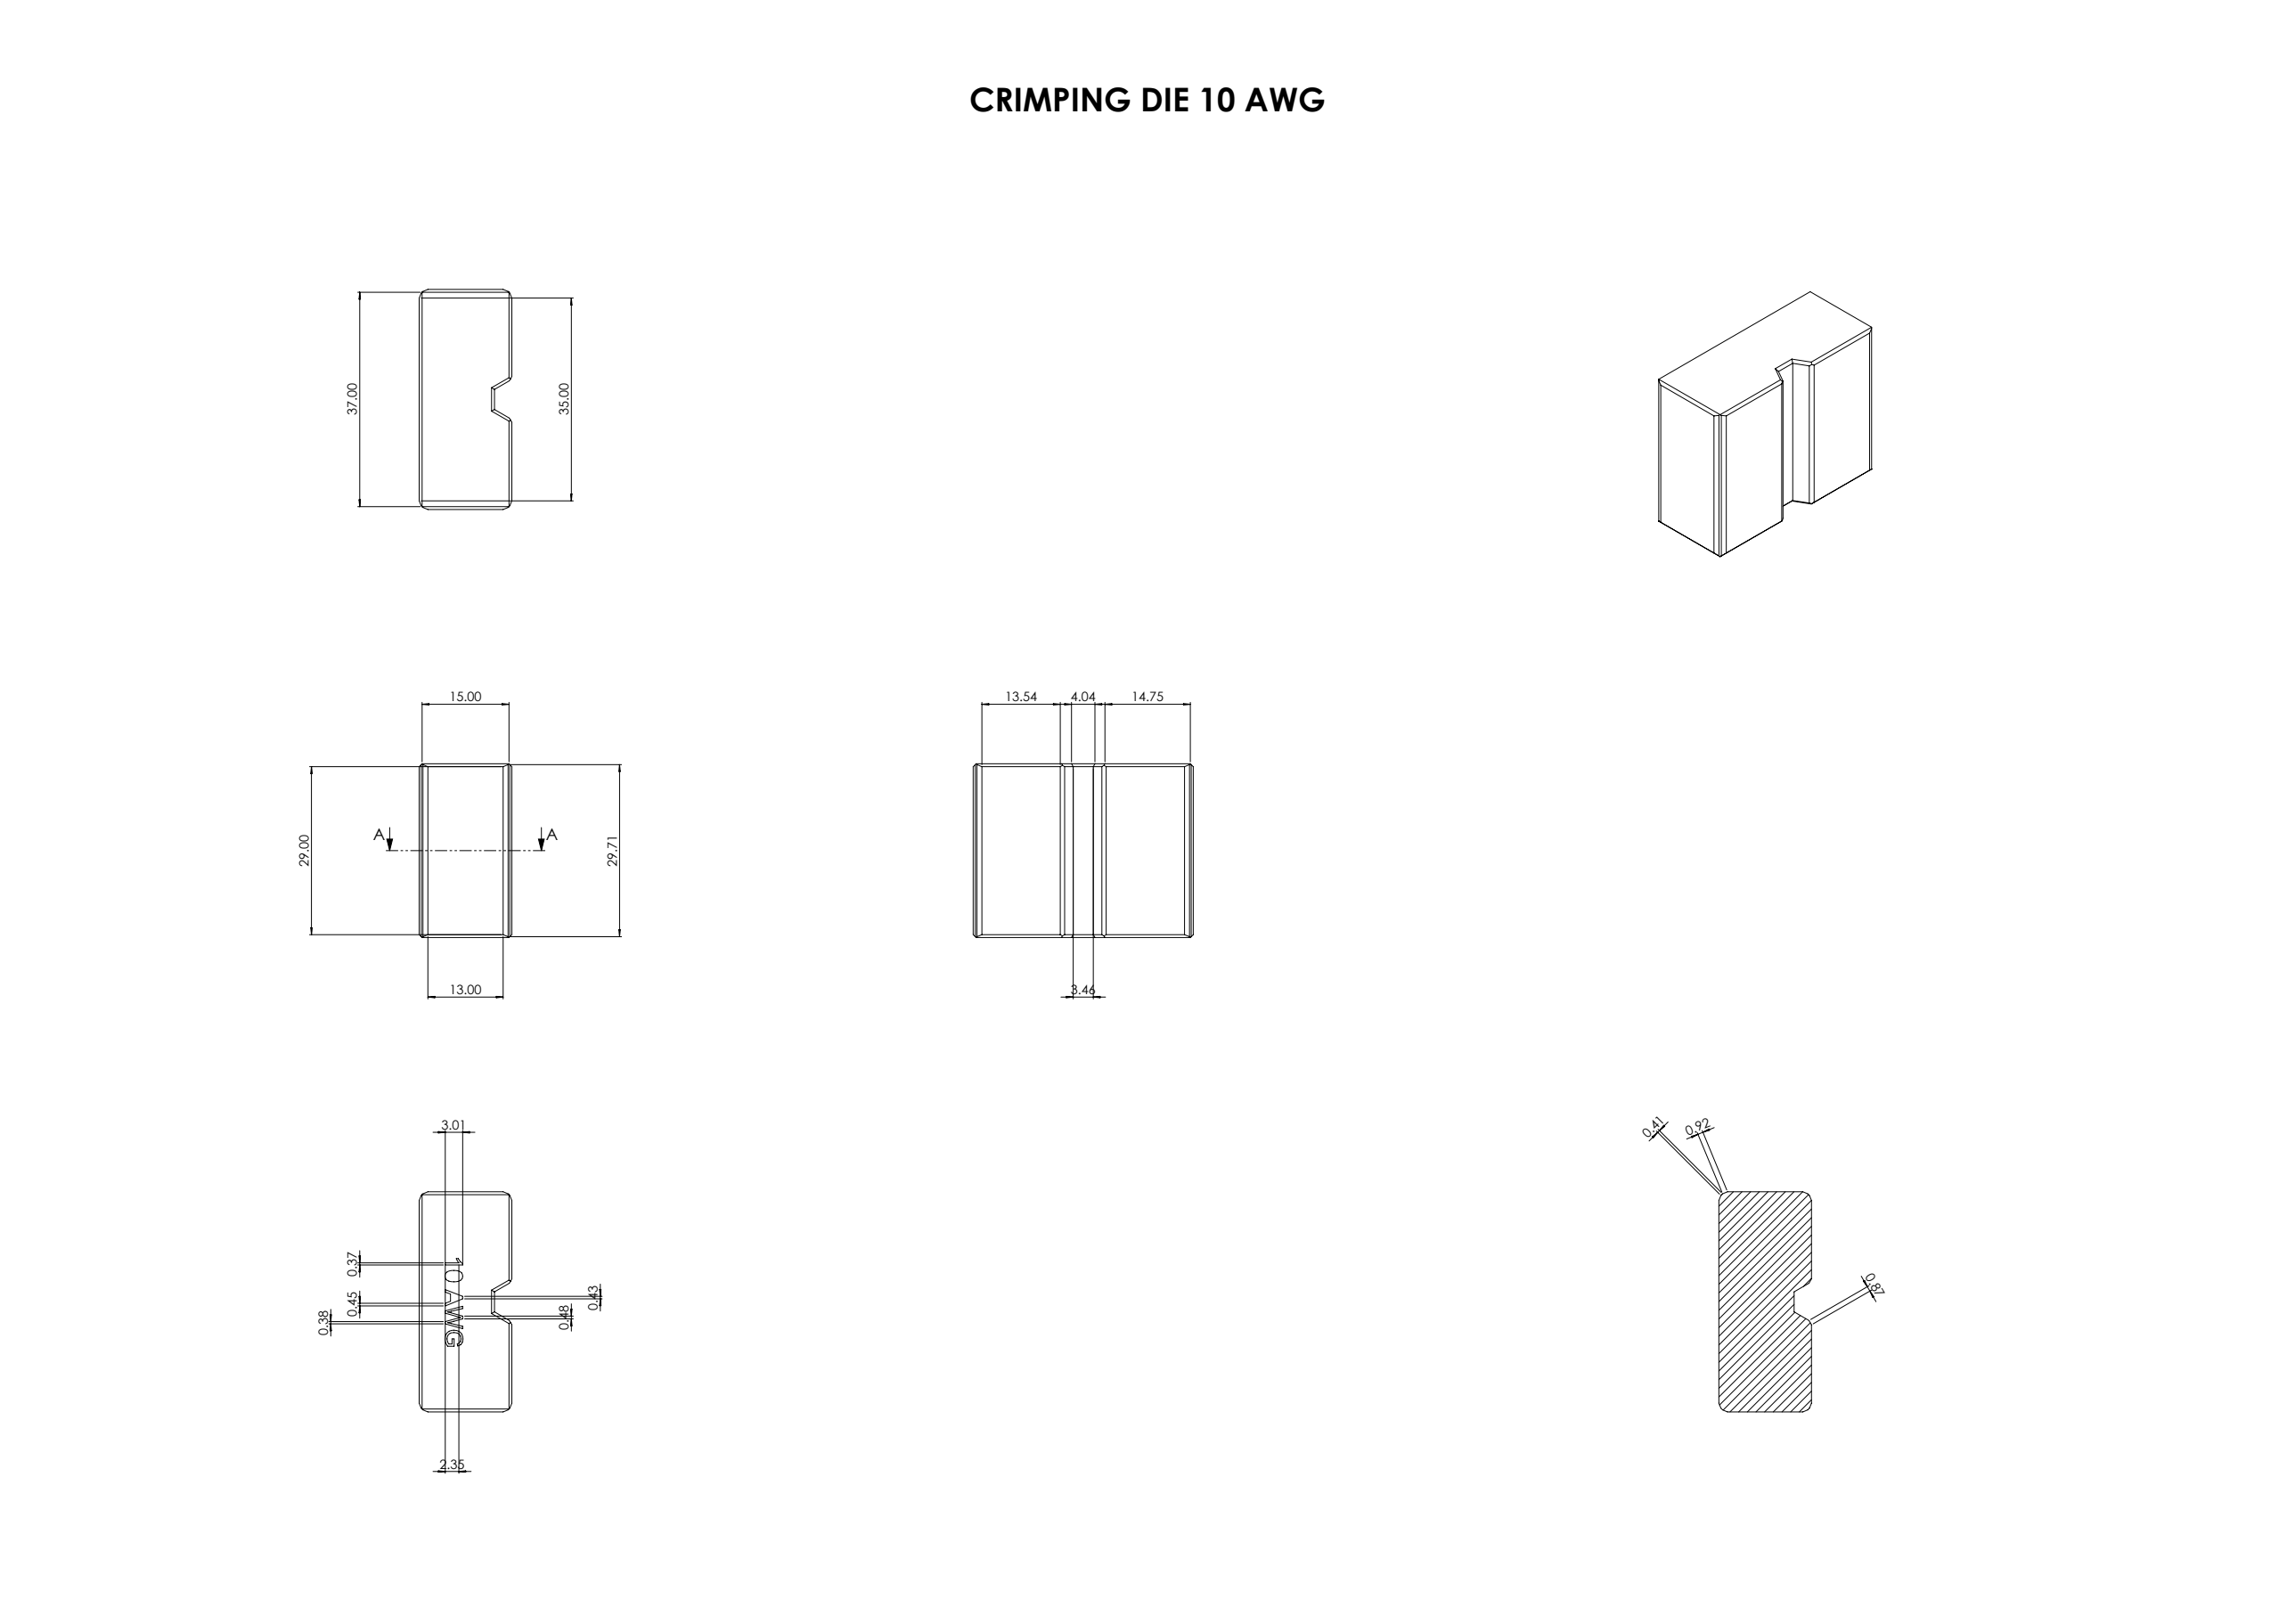
ISO-10303-21;
HEADER;
/* Generated by software containing ST-Developer
 * from STEP Tools, Inc. (www.steptools.com) 
 */

FILE_DESCRIPTION(
/* description */ (''),
/* implementation_level */ '2;1');

FILE_NAME(
/* name */ '08_Crimping_Die_10_AWG.step',
/* time_stamp */ '2026-10-26T03:55:20-07:00',
/* author */ (''),
/* organization */ (''),
/* preprocessor_version */ 'ST-DEVELOPER v20.2',
/* originating_system */ 'Autodesk Translation Framework v15.15.0.0',
/* authorisation */ '');

FILE_SCHEMA (('AUTOMOTIVE_DESIGN { 1 0 10303 214 3 1 1 }'));
ENDSEC;

DATA;
#10=MECHANICAL_DESIGN_GEOMETRIC_PRESENTATION_REPRESENTATION('',(#182),#45236);
#142=SHAPE_REPRESENTATION_RELATIONSHIP('SRR','None',#45321,#162);
#162=ADVANCED_BREP_SHAPE_REPRESENTATION('',(#202),#45223);
#182=STYLED_ITEM('',(#45477),#202);
#202=MANIFOLD_SOLID_BREP('Body1',#16524);
#485=B_SPLINE_CURVE_WITH_KNOTS('',2,(#32438,#32439,#32440),
 .UNSPECIFIED.,.F.,.F.,(3,3),(0.,1.),.UNSPECIFIED.);
#486=B_SPLINE_CURVE_WITH_KNOTS('',2,(#32452,#32453,#32454),
 .UNSPECIFIED.,.F.,.F.,(3,3),(0.,1.),.UNSPECIFIED.);
#487=B_SPLINE_CURVE_WITH_KNOTS('',2,(#32456,#32457,#32458),
 .UNSPECIFIED.,.F.,.F.,(3,3),(0.,1.),.UNSPECIFIED.);
#488=B_SPLINE_CURVE_WITH_KNOTS('',2,(#32466,#32467,#32468),
 .UNSPECIFIED.,.F.,.F.,(3,3),(0.,1.),.UNSPECIFIED.);
#489=B_SPLINE_CURVE_WITH_KNOTS('',2,(#32470,#32471,#32472),
 .UNSPECIFIED.,.F.,.F.,(3,3),(0.,1.),.UNSPECIFIED.);
#490=B_SPLINE_CURVE_WITH_KNOTS('',2,(#32483,#32484,#32485),
 .UNSPECIFIED.,.F.,.F.,(3,3),(0.,1.),.UNSPECIFIED.);
#491=B_SPLINE_CURVE_WITH_KNOTS('',2,(#32504,#32505,#32506),
 .UNSPECIFIED.,.F.,.F.,(3,3),(0.,1.),.UNSPECIFIED.);
#492=B_SPLINE_CURVE_WITH_KNOTS('',2,(#32508,#32509,#32510),
 .UNSPECIFIED.,.F.,.F.,(3,3),(0.,1.),.UNSPECIFIED.);
#493=B_SPLINE_CURVE_WITH_KNOTS('',2,(#32512,#32513,#32514),
 .UNSPECIFIED.,.F.,.F.,(3,3),(0.,1.),.UNSPECIFIED.);
#494=B_SPLINE_CURVE_WITH_KNOTS('',2,(#32516,#32517,#32518),
 .UNSPECIFIED.,.F.,.F.,(3,3),(0.,1.),.UNSPECIFIED.);
#495=B_SPLINE_CURVE_WITH_KNOTS('',2,(#32520,#32521,#32522),
 .UNSPECIFIED.,.F.,.F.,(3,3),(0.,1.),.UNSPECIFIED.);
#496=B_SPLINE_CURVE_WITH_KNOTS('',2,(#32524,#32525,#32526),
 .UNSPECIFIED.,.F.,.F.,(3,3),(0.,1.),.UNSPECIFIED.);
#497=B_SPLINE_CURVE_WITH_KNOTS('',2,(#32528,#32529,#32530),
 .UNSPECIFIED.,.F.,.F.,(3,3),(0.,1.),.UNSPECIFIED.);
#498=B_SPLINE_CURVE_WITH_KNOTS('',2,(#32532,#32533,#32534),
 .UNSPECIFIED.,.F.,.F.,(3,3),(0.,1.),.UNSPECIFIED.);
#499=B_SPLINE_CURVE_WITH_KNOTS('',2,(#32536,#32537,#32538),
 .UNSPECIFIED.,.F.,.F.,(3,3),(0.,1.),.UNSPECIFIED.);
#500=B_SPLINE_CURVE_WITH_KNOTS('',2,(#32540,#32541,#32542),
 .UNSPECIFIED.,.F.,.F.,(3,3),(0.,1.),.UNSPECIFIED.);
#501=B_SPLINE_CURVE_WITH_KNOTS('',2,(#32544,#32545,#32546),
 .UNSPECIFIED.,.F.,.F.,(3,3),(0.,1.),.UNSPECIFIED.);
#502=B_SPLINE_CURVE_WITH_KNOTS('',2,(#32547,#32548,#32549),
 .UNSPECIFIED.,.F.,.F.,(3,3),(0.,1.),.UNSPECIFIED.);
#503=B_SPLINE_CURVE_WITH_KNOTS('',2,(#32552,#32553,#32554),
 .UNSPECIFIED.,.F.,.F.,(3,3),(0.,1.),.UNSPECIFIED.);
#504=B_SPLINE_CURVE_WITH_KNOTS('',2,(#32564,#32565,#32566),
 .UNSPECIFIED.,.F.,.F.,(3,3),(0.,1.),.UNSPECIFIED.);
#505=B_SPLINE_CURVE_WITH_KNOTS('',2,(#32568,#32569,#32570),
 .UNSPECIFIED.,.F.,.F.,(3,3),(0.,1.),.UNSPECIFIED.);
#506=B_SPLINE_CURVE_WITH_KNOTS('',2,(#32573,#32574,#32575),
 .UNSPECIFIED.,.F.,.F.,(3,3),(0.,1.),.UNSPECIFIED.);
#507=B_SPLINE_CURVE_WITH_KNOTS('',2,(#32578,#32579,#32580),
 .UNSPECIFIED.,.F.,.F.,(3,3),(0.,1.),.UNSPECIFIED.);
#508=B_SPLINE_CURVE_WITH_KNOTS('',2,(#32592,#32593,#32594),
 .UNSPECIFIED.,.F.,.F.,(3,3),(0.,1.),.UNSPECIFIED.);
#509=B_SPLINE_CURVE_WITH_KNOTS('',2,(#32596,#32597,#32598),
 .UNSPECIFIED.,.F.,.F.,(3,3),(0.,1.),.UNSPECIFIED.);
#510=B_SPLINE_CURVE_WITH_KNOTS('',2,(#32600,#32601,#32602),
 .UNSPECIFIED.,.F.,.F.,(3,3),(0.,1.),.UNSPECIFIED.);
#511=B_SPLINE_CURVE_WITH_KNOTS('',2,(#32604,#32605,#32606),
 .UNSPECIFIED.,.F.,.F.,(3,3),(0.,1.),.UNSPECIFIED.);
#512=B_SPLINE_CURVE_WITH_KNOTS('',2,(#32608,#32609,#32610),
 .UNSPECIFIED.,.F.,.F.,(3,3),(0.,1.),.UNSPECIFIED.);
#513=B_SPLINE_CURVE_WITH_KNOTS('',2,(#32612,#32613,#32614),
 .UNSPECIFIED.,.F.,.F.,(3,3),(0.,1.),.UNSPECIFIED.);
#514=B_SPLINE_CURVE_WITH_KNOTS('',2,(#32616,#32617,#32618),
 .UNSPECIFIED.,.F.,.F.,(3,3),(0.,1.),.UNSPECIFIED.);
#515=B_SPLINE_CURVE_WITH_KNOTS('',2,(#32620,#32621,#32622),
 .UNSPECIFIED.,.F.,.F.,(3,3),(0.,1.),.UNSPECIFIED.);
#516=B_SPLINE_CURVE_WITH_KNOTS('',2,(#32624,#32625,#32626),
 .UNSPECIFIED.,.F.,.F.,(3,3),(0.,1.),.UNSPECIFIED.);
#517=B_SPLINE_CURVE_WITH_KNOTS('',2,(#32628,#32629,#32630),
 .UNSPECIFIED.,.F.,.F.,(3,3),(0.,1.),.UNSPECIFIED.);
#518=B_SPLINE_CURVE_WITH_KNOTS('',2,(#32632,#32633,#32634),
 .UNSPECIFIED.,.F.,.F.,(3,3),(0.,1.),.UNSPECIFIED.);
#519=B_SPLINE_CURVE_WITH_KNOTS('',2,(#32638,#32639,#32640),
 .UNSPECIFIED.,.F.,.F.,(3,3),(0.,1.),.UNSPECIFIED.);
#520=B_SPLINE_CURVE_WITH_KNOTS('',2,(#32642,#32643,#32644),
 .UNSPECIFIED.,.F.,.F.,(3,3),(0.,1.),.UNSPECIFIED.);
#521=B_SPLINE_CURVE_WITH_KNOTS('',2,(#32646,#32647,#32648),
 .UNSPECIFIED.,.F.,.F.,(3,3),(0.,1.),.UNSPECIFIED.);
#522=B_SPLINE_CURVE_WITH_KNOTS('',2,(#32650,#32651,#32652),
 .UNSPECIFIED.,.F.,.F.,(3,3),(0.,1.),.UNSPECIFIED.);
#523=B_SPLINE_CURVE_WITH_KNOTS('',2,(#32654,#32655,#32656),
 .UNSPECIFIED.,.F.,.F.,(3,3),(0.,1.),.UNSPECIFIED.);
#524=B_SPLINE_CURVE_WITH_KNOTS('',2,(#32658,#32659,#32660),
 .UNSPECIFIED.,.F.,.F.,(3,3),(0.,1.),.UNSPECIFIED.);
#525=B_SPLINE_CURVE_WITH_KNOTS('',2,(#32662,#32663,#32664),
 .UNSPECIFIED.,.F.,.F.,(3,3),(0.,1.),.UNSPECIFIED.);
#526=B_SPLINE_CURVE_WITH_KNOTS('',2,(#32666,#32667,#32668),
 .UNSPECIFIED.,.F.,.F.,(3,3),(0.,1.),.UNSPECIFIED.);
#527=B_SPLINE_CURVE_WITH_KNOTS('',2,(#32670,#32671,#32672),
 .UNSPECIFIED.,.F.,.F.,(3,3),(0.,1.),.UNSPECIFIED.);
#528=B_SPLINE_CURVE_WITH_KNOTS('',2,(#32674,#32675,#32676),
 .UNSPECIFIED.,.F.,.F.,(3,3),(0.,1.),.UNSPECIFIED.);
#529=B_SPLINE_CURVE_WITH_KNOTS('',2,(#32677,#32678,#32679),
 .UNSPECIFIED.,.F.,.F.,(3,3),(0.,1.),.UNSPECIFIED.);
#530=B_SPLINE_CURVE_WITH_KNOTS('',2,(#32712,#32713,#32714),
 .UNSPECIFIED.,.F.,.F.,(3,3),(0.,1.),.UNSPECIFIED.);
#531=B_SPLINE_CURVE_WITH_KNOTS('',2,(#32724,#32725,#32726),
 .UNSPECIFIED.,.F.,.F.,(3,3),(0.,1.),.UNSPECIFIED.);
#532=B_SPLINE_CURVE_WITH_KNOTS('',2,(#32755,#32756,#32757),
 .UNSPECIFIED.,.F.,.F.,(3,3),(0.,1.),.UNSPECIFIED.);
#533=B_SPLINE_CURVE_WITH_KNOTS('',2,(#32766,#32767,#32768),
 .UNSPECIFIED.,.F.,.F.,(3,3),(0.,1.),.UNSPECIFIED.);
#534=B_SPLINE_CURVE_WITH_KNOTS('',2,(#32789,#32790,#32791),
 .UNSPECIFIED.,.F.,.F.,(3,3),(0.,1.),.UNSPECIFIED.);
#535=B_SPLINE_CURVE_WITH_KNOTS('',2,(#32800,#32801,#32802),
 .UNSPECIFIED.,.F.,.F.,(3,3),(0.,1.),.UNSPECIFIED.);
#536=B_SPLINE_CURVE_WITH_KNOTS('',2,(#32864,#32865,#32866),
 .UNSPECIFIED.,.F.,.F.,(3,3),(0.,1.),.UNSPECIFIED.);
#537=B_SPLINE_CURVE_WITH_KNOTS('',2,(#32876,#32877,#32878),
 .UNSPECIFIED.,.F.,.F.,(3,3),(0.,1.),.UNSPECIFIED.);
#538=B_SPLINE_CURVE_WITH_KNOTS('',2,(#32887,#32888,#32889),
 .UNSPECIFIED.,.F.,.F.,(3,3),(0.,1.),.UNSPECIFIED.);
#539=B_SPLINE_CURVE_WITH_KNOTS('',2,(#32898,#32899,#32900),
 .UNSPECIFIED.,.F.,.F.,(3,3),(0.,1.),.UNSPECIFIED.);
#540=B_SPLINE_CURVE_WITH_KNOTS('',2,(#32909,#32910,#32911),
 .UNSPECIFIED.,.F.,.F.,(3,3),(0.,1.),.UNSPECIFIED.);
#541=B_SPLINE_CURVE_WITH_KNOTS('',2,(#32920,#32921,#32922),
 .UNSPECIFIED.,.F.,.F.,(3,3),(0.,1.),.UNSPECIFIED.);
#542=B_SPLINE_CURVE_WITH_KNOTS('',2,(#32931,#32932,#32933),
 .UNSPECIFIED.,.F.,.F.,(3,3),(0.,1.),.UNSPECIFIED.);
#543=B_SPLINE_CURVE_WITH_KNOTS('',2,(#32942,#32943,#32944),
 .UNSPECIFIED.,.F.,.F.,(3,3),(0.,1.),.UNSPECIFIED.);
#544=B_SPLINE_CURVE_WITH_KNOTS('',2,(#32953,#32954,#32955),
 .UNSPECIFIED.,.F.,.F.,(3,3),(0.,1.),.UNSPECIFIED.);
#545=B_SPLINE_CURVE_WITH_KNOTS('',2,(#32964,#32965,#32966),
 .UNSPECIFIED.,.F.,.F.,(3,3),(0.,1.),.UNSPECIFIED.);
#546=B_SPLINE_CURVE_WITH_KNOTS('',2,(#32975,#32976,#32977),
 .UNSPECIFIED.,.F.,.F.,(3,3),(0.,1.),.UNSPECIFIED.);
#547=B_SPLINE_CURVE_WITH_KNOTS('',2,(#32984,#32985,#32986),
 .UNSPECIFIED.,.F.,.F.,(3,3),(0.,1.),.UNSPECIFIED.);
#548=B_SPLINE_CURVE_WITH_KNOTS('',2,(#32997,#32998,#32999),
 .UNSPECIFIED.,.F.,.F.,(3,3),(0.,1.),.UNSPECIFIED.);
#549=B_SPLINE_CURVE_WITH_KNOTS('',2,(#33009,#33010,#33011),
 .UNSPECIFIED.,.F.,.F.,(3,3),(0.,1.),.UNSPECIFIED.);
#550=B_SPLINE_CURVE_WITH_KNOTS('',2,(#33024,#33025,#33026),
 .UNSPECIFIED.,.F.,.F.,(3,3),(0.,1.),.UNSPECIFIED.);
#551=B_SPLINE_CURVE_WITH_KNOTS('',2,(#33035,#33036,#33037),
 .UNSPECIFIED.,.F.,.F.,(3,3),(0.,1.),.UNSPECIFIED.);
#552=B_SPLINE_CURVE_WITH_KNOTS('',2,(#33062,#33063,#33064),
 .UNSPECIFIED.,.F.,.F.,(3,3),(0.,1.),.UNSPECIFIED.);
#553=B_SPLINE_CURVE_WITH_KNOTS('',2,(#33074,#33075,#33076),
 .UNSPECIFIED.,.F.,.F.,(3,3),(0.,1.),.UNSPECIFIED.);
#554=B_SPLINE_CURVE_WITH_KNOTS('',2,(#33085,#33086,#33087),
 .UNSPECIFIED.,.F.,.F.,(3,3),(0.,1.),.UNSPECIFIED.);
#555=B_SPLINE_CURVE_WITH_KNOTS('',2,(#33096,#33097,#33098),
 .UNSPECIFIED.,.F.,.F.,(3,3),(0.,1.),.UNSPECIFIED.);
#556=B_SPLINE_CURVE_WITH_KNOTS('',2,(#33107,#33108,#33109),
 .UNSPECIFIED.,.F.,.F.,(3,3),(0.,1.),.UNSPECIFIED.);
#557=B_SPLINE_CURVE_WITH_KNOTS('',2,(#33118,#33119,#33120),
 .UNSPECIFIED.,.F.,.F.,(3,3),(0.,1.),.UNSPECIFIED.);
#558=B_SPLINE_CURVE_WITH_KNOTS('',2,(#33129,#33130,#33131),
 .UNSPECIFIED.,.F.,.F.,(3,3),(0.,1.),.UNSPECIFIED.);
#559=B_SPLINE_CURVE_WITH_KNOTS('',2,(#33140,#33141,#33142),
 .UNSPECIFIED.,.F.,.F.,(3,3),(0.,1.),.UNSPECIFIED.);
#560=B_SPLINE_CURVE_WITH_KNOTS('',2,(#33151,#33152,#33153),
 .UNSPECIFIED.,.F.,.F.,(3,3),(0.,1.),.UNSPECIFIED.);
#561=B_SPLINE_CURVE_WITH_KNOTS('',2,(#33162,#33163,#33164),
 .UNSPECIFIED.,.F.,.F.,(3,3),(0.,1.),.UNSPECIFIED.);
#562=B_SPLINE_CURVE_WITH_KNOTS('',2,(#33173,#33174,#33175),
 .UNSPECIFIED.,.F.,.F.,(3,3),(0.,1.),.UNSPECIFIED.);
#563=B_SPLINE_CURVE_WITH_KNOTS('',2,(#33184,#33185,#33186),
 .UNSPECIFIED.,.F.,.F.,(3,3),(0.,1.),.UNSPECIFIED.);
#564=B_SPLINE_CURVE_WITH_KNOTS('',2,(#33199,#33200,#33201),
 .UNSPECIFIED.,.F.,.F.,(3,3),(0.,1.),.UNSPECIFIED.);
#565=B_SPLINE_CURVE_WITH_KNOTS('',2,(#33210,#33211,#33212),
 .UNSPECIFIED.,.F.,.F.,(3,3),(0.,1.),.UNSPECIFIED.);
#566=B_SPLINE_CURVE_WITH_KNOTS('',2,(#33221,#33222,#33223),
 .UNSPECIFIED.,.F.,.F.,(3,3),(0.,1.),.UNSPECIFIED.);
#567=B_SPLINE_CURVE_WITH_KNOTS('',2,(#33232,#33233,#33234),
 .UNSPECIFIED.,.F.,.F.,(3,3),(0.,1.),.UNSPECIFIED.);
#568=B_SPLINE_CURVE_WITH_KNOTS('',2,(#33243,#33244,#33245),
 .UNSPECIFIED.,.F.,.F.,(3,3),(0.,1.),.UNSPECIFIED.);
#569=B_SPLINE_CURVE_WITH_KNOTS('',2,(#33254,#33255,#33256),
 .UNSPECIFIED.,.F.,.F.,(3,3),(0.,1.),.UNSPECIFIED.);
#570=B_SPLINE_CURVE_WITH_KNOTS('',2,(#33265,#33266,#33267),
 .UNSPECIFIED.,.F.,.F.,(3,3),(0.,1.),.UNSPECIFIED.);
#571=B_SPLINE_CURVE_WITH_KNOTS('',2,(#33276,#33277,#33278),
 .UNSPECIFIED.,.F.,.F.,(3,3),(0.,1.),.UNSPECIFIED.);
#572=B_SPLINE_CURVE_WITH_KNOTS('',2,(#33287,#33288,#33289),
 .UNSPECIFIED.,.F.,.F.,(3,3),(0.,1.),.UNSPECIFIED.);
#573=B_SPLINE_CURVE_WITH_KNOTS('',2,(#33298,#33299,#33300),
 .UNSPECIFIED.,.F.,.F.,(3,3),(0.,1.),.UNSPECIFIED.);
#574=B_SPLINE_CURVE_WITH_KNOTS('',2,(#33309,#33310,#33311),
 .UNSPECIFIED.,.F.,.F.,(3,3),(0.,1.),.UNSPECIFIED.);
#858=B_SPLINE_SURFACE_WITH_KNOTS('',2,1,((#32703,#32704),(#32705,#32706),
(#32707,#32708)),.UNSPECIFIED.,.F.,.F.,.F.,(3,3),(2,2),(0.,1.),(0.,0.0249999999999999),
 .UNSPECIFIED.);
#859=B_SPLINE_SURFACE_WITH_KNOTS('',2,1,((#32716,#32717),(#32718,#32719),
(#32720,#32721)),.UNSPECIFIED.,.F.,.F.,.F.,(3,3),(2,2),(0.,1.),(0.,0.0249999999999999),
 .UNSPECIFIED.);
#860=B_SPLINE_SURFACE_WITH_KNOTS('',2,1,((#32747,#32748),(#32749,#32750),
(#32751,#32752)),.UNSPECIFIED.,.F.,.F.,.F.,(3,3),(2,2),(0.,1.),(0.,0.0249999999999999),
 .UNSPECIFIED.);
#861=B_SPLINE_SURFACE_WITH_KNOTS('',2,1,((#32758,#32759),(#32760,#32761),
(#32762,#32763)),.UNSPECIFIED.,.F.,.F.,.F.,(3,3),(2,2),(0.,1.),(0.,0.0249999999999999),
 .UNSPECIFIED.);
#862=B_SPLINE_SURFACE_WITH_KNOTS('',2,1,((#32781,#32782),(#32783,#32784),
(#32785,#32786)),.UNSPECIFIED.,.F.,.F.,.F.,(3,3),(2,2),(0.,1.),(0.,0.0249999999999999),
 .UNSPECIFIED.);
#863=B_SPLINE_SURFACE_WITH_KNOTS('',2,1,((#32792,#32793),(#32794,#32795),
(#32796,#32797)),.UNSPECIFIED.,.F.,.F.,.F.,(3,3),(2,2),(0.,1.),(0.,0.0249999999999999),
 .UNSPECIFIED.);
#864=B_SPLINE_SURFACE_WITH_KNOTS('',2,1,((#32855,#32856),(#32857,#32858),
(#32859,#32860)),.UNSPECIFIED.,.F.,.F.,.F.,(3,3),(2,2),(0.,1.),(0.,0.0249999999999999),
 .UNSPECIFIED.);
#865=B_SPLINE_SURFACE_WITH_KNOTS('',2,1,((#32868,#32869),(#32870,#32871),
(#32872,#32873)),.UNSPECIFIED.,.F.,.F.,.F.,(3,3),(2,2),(0.,1.),(0.,0.0249999999999999),
 .UNSPECIFIED.);
#866=B_SPLINE_SURFACE_WITH_KNOTS('',2,1,((#32879,#32880),(#32881,#32882),
(#32883,#32884)),.UNSPECIFIED.,.F.,.F.,.F.,(3,3),(2,2),(0.,1.),(0.,0.0249999999999999),
 .UNSPECIFIED.);
#867=B_SPLINE_SURFACE_WITH_KNOTS('',2,1,((#32890,#32891),(#32892,#32893),
(#32894,#32895)),.UNSPECIFIED.,.F.,.F.,.F.,(3,3),(2,2),(0.,1.),(0.,0.0249999999999999),
 .UNSPECIFIED.);
#868=B_SPLINE_SURFACE_WITH_KNOTS('',2,1,((#32901,#32902),(#32903,#32904),
(#32905,#32906)),.UNSPECIFIED.,.F.,.F.,.F.,(3,3),(2,2),(0.,1.),(0.,0.0249999999999999),
 .UNSPECIFIED.);
#869=B_SPLINE_SURFACE_WITH_KNOTS('',2,1,((#32912,#32913),(#32914,#32915),
(#32916,#32917)),.UNSPECIFIED.,.F.,.F.,.F.,(3,3),(2,2),(0.,1.),(0.,0.0249999999999999),
 .UNSPECIFIED.);
#870=B_SPLINE_SURFACE_WITH_KNOTS('',2,1,((#32923,#32924),(#32925,#32926),
(#32927,#32928)),.UNSPECIFIED.,.F.,.F.,.F.,(3,3),(2,2),(0.,1.),(0.,0.0249999999999999),
 .UNSPECIFIED.);
#871=B_SPLINE_SURFACE_WITH_KNOTS('',2,1,((#32934,#32935),(#32936,#32937),
(#32938,#32939)),.UNSPECIFIED.,.F.,.F.,.F.,(3,3),(2,2),(0.,1.),(0.,0.0249999999999999),
 .UNSPECIFIED.);
#872=B_SPLINE_SURFACE_WITH_KNOTS('',2,1,((#32945,#32946),(#32947,#32948),
(#32949,#32950)),.UNSPECIFIED.,.F.,.F.,.F.,(3,3),(2,2),(0.,1.),(0.,0.0249999999999999),
 .UNSPECIFIED.);
#873=B_SPLINE_SURFACE_WITH_KNOTS('',2,1,((#32956,#32957),(#32958,#32959),
(#32960,#32961)),.UNSPECIFIED.,.F.,.F.,.F.,(3,3),(2,2),(0.,1.),(0.,0.0249999999999999),
 .UNSPECIFIED.);
#874=B_SPLINE_SURFACE_WITH_KNOTS('',2,1,((#32967,#32968),(#32969,#32970),
(#32971,#32972)),.UNSPECIFIED.,.F.,.F.,.F.,(3,3),(2,2),(0.,1.),(0.,0.0249999999999999),
 .UNSPECIFIED.);
#875=B_SPLINE_SURFACE_WITH_KNOTS('',2,1,((#32978,#32979),(#32980,#32981),
(#32982,#32983)),.UNSPECIFIED.,.F.,.F.,.F.,(3,3),(2,2),(0.,1.),(0.,0.0249999999999999),
 .UNSPECIFIED.);
#876=B_SPLINE_SURFACE_WITH_KNOTS('',2,1,((#32988,#32989),(#32990,#32991),
(#32992,#32993)),.UNSPECIFIED.,.F.,.F.,.F.,(3,3),(2,2),(0.,1.),(0.,0.0249999999999999),
 .UNSPECIFIED.);
#877=B_SPLINE_SURFACE_WITH_KNOTS('',2,1,((#33001,#33002),(#33003,#33004),
(#33005,#33006)),.UNSPECIFIED.,.F.,.F.,.F.,(3,3),(2,2),(0.,1.),(0.,0.0249999999999999),
 .UNSPECIFIED.);
#878=B_SPLINE_SURFACE_WITH_KNOTS('',2,1,((#33016,#33017),(#33018,#33019),
(#33020,#33021)),.UNSPECIFIED.,.F.,.F.,.F.,(3,3),(2,2),(0.,1.),(0.,0.0249999999999999),
 .UNSPECIFIED.);
#879=B_SPLINE_SURFACE_WITH_KNOTS('',2,1,((#33027,#33028),(#33029,#33030),
(#33031,#33032)),.UNSPECIFIED.,.F.,.F.,.F.,(3,3),(2,2),(0.,1.),(0.,0.0249999999999999),
 .UNSPECIFIED.);
#880=B_SPLINE_SURFACE_WITH_KNOTS('',2,1,((#33053,#33054),(#33055,#33056),
(#33057,#33058)),.UNSPECIFIED.,.F.,.F.,.F.,(3,3),(2,2),(0.,1.),(0.,0.0249999999999999),
 .UNSPECIFIED.);
#881=B_SPLINE_SURFACE_WITH_KNOTS('',2,1,((#33066,#33067),(#33068,#33069),
(#33070,#33071)),.UNSPECIFIED.,.F.,.F.,.F.,(3,3),(2,2),(0.,1.),(0.,0.0249999999999999),
 .UNSPECIFIED.);
#882=B_SPLINE_SURFACE_WITH_KNOTS('',2,1,((#33077,#33078),(#33079,#33080),
(#33081,#33082)),.UNSPECIFIED.,.F.,.F.,.F.,(3,3),(2,2),(0.,1.),(0.,0.0249999999999999),
 .UNSPECIFIED.);
#883=B_SPLINE_SURFACE_WITH_KNOTS('',2,1,((#33088,#33089),(#33090,#33091),
(#33092,#33093)),.UNSPECIFIED.,.F.,.F.,.F.,(3,3),(2,2),(0.,1.),(0.,0.0249999999999999),
 .UNSPECIFIED.);
#884=B_SPLINE_SURFACE_WITH_KNOTS('',2,1,((#33099,#33100),(#33101,#33102),
(#33103,#33104)),.UNSPECIFIED.,.F.,.F.,.F.,(3,3),(2,2),(0.,1.),(0.,0.0249999999999999),
 .UNSPECIFIED.);
#885=B_SPLINE_SURFACE_WITH_KNOTS('',2,1,((#33110,#33111),(#33112,#33113),
(#33114,#33115)),.UNSPECIFIED.,.F.,.F.,.F.,(3,3),(2,2),(0.,1.),(0.,0.0249999999999999),
 .UNSPECIFIED.);
#886=B_SPLINE_SURFACE_WITH_KNOTS('',2,1,((#33121,#33122),(#33123,#33124),
(#33125,#33126)),.UNSPECIFIED.,.F.,.F.,.F.,(3,3),(2,2),(0.,1.),(0.,0.0249999999999999),
 .UNSPECIFIED.);
#887=B_SPLINE_SURFACE_WITH_KNOTS('',2,1,((#33132,#33133),(#33134,#33135),
(#33136,#33137)),.UNSPECIFIED.,.F.,.F.,.F.,(3,3),(2,2),(0.,1.),(0.,0.0249999999999999),
 .UNSPECIFIED.);
#888=B_SPLINE_SURFACE_WITH_KNOTS('',2,1,((#33143,#33144),(#33145,#33146),
(#33147,#33148)),.UNSPECIFIED.,.F.,.F.,.F.,(3,3),(2,2),(0.,1.),(0.,0.0249999999999999),
 .UNSPECIFIED.);
#889=B_SPLINE_SURFACE_WITH_KNOTS('',2,1,((#33154,#33155),(#33156,#33157),
(#33158,#33159)),.UNSPECIFIED.,.F.,.F.,.F.,(3,3),(2,2),(0.,1.),(0.,0.0249999999999999),
 .UNSPECIFIED.);
#890=B_SPLINE_SURFACE_WITH_KNOTS('',2,1,((#33165,#33166),(#33167,#33168),
(#33169,#33170)),.UNSPECIFIED.,.F.,.F.,.F.,(3,3),(2,2),(0.,1.),(0.,0.0249999999999999),
 .UNSPECIFIED.);
#891=B_SPLINE_SURFACE_WITH_KNOTS('',2,1,((#33176,#33177),(#33178,#33179),
(#33180,#33181)),.UNSPECIFIED.,.F.,.F.,.F.,(3,3),(2,2),(0.,1.),(0.,0.0249999999999999),
 .UNSPECIFIED.);
#892=B_SPLINE_SURFACE_WITH_KNOTS('',2,1,((#33191,#33192),(#33193,#33194),
(#33195,#33196)),.UNSPECIFIED.,.F.,.F.,.F.,(3,3),(2,2),(0.,1.),(0.,0.0249999999999999),
 .UNSPECIFIED.);
#893=B_SPLINE_SURFACE_WITH_KNOTS('',2,1,((#33202,#33203),(#33204,#33205),
(#33206,#33207)),.UNSPECIFIED.,.F.,.F.,.F.,(3,3),(2,2),(0.,1.),(0.,0.0249999999999999),
 .UNSPECIFIED.);
#894=B_SPLINE_SURFACE_WITH_KNOTS('',2,1,((#33213,#33214),(#33215,#33216),
(#33217,#33218)),.UNSPECIFIED.,.F.,.F.,.F.,(3,3),(2,2),(0.,1.),(0.,0.0249999999999999),
 .UNSPECIFIED.);
#895=B_SPLINE_SURFACE_WITH_KNOTS('',2,1,((#33224,#33225),(#33226,#33227),
(#33228,#33229)),.UNSPECIFIED.,.F.,.F.,.F.,(3,3),(2,2),(0.,1.),(0.,0.0249999999999999),
 .UNSPECIFIED.);
#896=B_SPLINE_SURFACE_WITH_KNOTS('',2,1,((#33235,#33236),(#33237,#33238),
(#33239,#33240)),.UNSPECIFIED.,.F.,.F.,.F.,(3,3),(2,2),(0.,1.),(0.,0.0249999999999999),
 .UNSPECIFIED.);
#897=B_SPLINE_SURFACE_WITH_KNOTS('',2,1,((#33246,#33247),(#33248,#33249),
(#33250,#33251)),.UNSPECIFIED.,.F.,.F.,.F.,(3,3),(2,2),(0.,1.),(0.,0.0249999999999999),
 .UNSPECIFIED.);
#898=B_SPLINE_SURFACE_WITH_KNOTS('',2,1,((#33257,#33258),(#33259,#33260),
(#33261,#33262)),.UNSPECIFIED.,.F.,.F.,.F.,(3,3),(2,2),(0.,1.),(0.,0.0249999999999999),
 .UNSPECIFIED.);
#899=B_SPLINE_SURFACE_WITH_KNOTS('',2,1,((#33268,#33269),(#33270,#33271),
(#33272,#33273)),.UNSPECIFIED.,.F.,.F.,.F.,(3,3),(2,2),(0.,1.),(0.,0.0249999999999999),
 .UNSPECIFIED.);
#900=B_SPLINE_SURFACE_WITH_KNOTS('',2,1,((#33279,#33280),(#33281,#33282),
(#33283,#33284)),.UNSPECIFIED.,.F.,.F.,.F.,(3,3),(2,2),(0.,1.),(0.,0.0249999999999999),
 .UNSPECIFIED.);
#901=B_SPLINE_SURFACE_WITH_KNOTS('',2,1,((#33290,#33291),(#33292,#33293),
(#33294,#33295)),.UNSPECIFIED.,.F.,.F.,.F.,(3,3),(2,2),(0.,1.),(0.,0.0249999999999999),
 .UNSPECIFIED.);
#902=B_SPLINE_SURFACE_WITH_KNOTS('',2,1,((#33301,#33302),(#33303,#33304),
(#33305,#33306)),.UNSPECIFIED.,.F.,.F.,.F.,(3,3),(2,2),(0.,1.),(0.,0.0249999999999999),
 .UNSPECIFIED.);
#965=FACE_BOUND('',#3127,.T.);
#966=FACE_BOUND('',#3128,.T.);
#967=FACE_BOUND('',#3129,.T.);
#968=FACE_BOUND('',#3130,.T.);
#969=FACE_BOUND('',#3131,.T.);
#1136=PLANE('',#17176);
#1137=PLANE('',#17177);
#1138=PLANE('',#17178);
#1139=PLANE('',#17179);
#1140=PLANE('',#17180);
#1141=PLANE('',#17181);
#1142=PLANE('',#17182);
#1143=PLANE('',#17183);
#1144=PLANE('',#17184);
#1145=PLANE('',#17185);
#1146=PLANE('',#17186);
#1147=PLANE('',#17187);
#1148=PLANE('',#17188);
#1149=PLANE('',#17189);
#1150=PLANE('',#17190);
#1151=PLANE('',#17191);
#1152=PLANE('',#17192);
#1153=PLANE('',#17193);
#1154=PLANE('',#17194);
#1155=PLANE('',#17195);
#1156=PLANE('',#17196);
#1157=PLANE('',#17197);
#1158=PLANE('',#17198);
#1159=PLANE('',#17199);
#1160=PLANE('',#17200);
#1161=PLANE('',#17201);
#1162=PLANE('',#17202);
#1163=PLANE('',#17203);
#1164=PLANE('',#17204);
#1165=PLANE('',#17205);
#1166=PLANE('',#17206);
#1167=PLANE('',#17207);
#1168=PLANE('',#17208);
#1169=PLANE('',#17209);
#1170=PLANE('',#17210);
#1171=PLANE('',#17211);
#1172=PLANE('',#17212);
#1173=PLANE('',#17213);
#1174=PLANE('',#17214);
#1175=PLANE('',#17215);
#1176=PLANE('',#17216);
#1177=PLANE('',#17217);
#1178=PLANE('',#17218);
#1179=PLANE('',#17219);
#1180=PLANE('',#17220);
#1181=PLANE('',#17221);
#1182=PLANE('',#17222);
#1183=PLANE('',#17223);
#1184=PLANE('',#17224);
#1185=PLANE('',#17225);
#1186=PLANE('',#17226);
#1187=PLANE('',#17227);
#1188=PLANE('',#17228);
#1189=PLANE('',#17229);
#1190=PLANE('',#17230);
#1191=PLANE('',#17231);
#1192=PLANE('',#17232);
#1193=PLANE('',#17233);
#1194=PLANE('',#17234);
#1195=PLANE('',#17235);
#1196=PLANE('',#17236);
#1197=PLANE('',#17237);
#1198=PLANE('',#17238);
#1199=PLANE('',#17239);
#1200=PLANE('',#17240);
#1201=PLANE('',#17241);
#1202=PLANE('',#17242);
#1203=PLANE('',#17243);
#1204=PLANE('',#17244);
#1205=PLANE('',#17245);
#1206=PLANE('',#17246);
#1207=PLANE('',#17247);
#1208=PLANE('',#17248);
#1209=PLANE('',#17249);
#1210=PLANE('',#17250);
#1211=PLANE('',#17251);
#1212=PLANE('',#17252);
#2101=FACE_OUTER_BOUND('',#3101,.T.);
#2102=FACE_OUTER_BOUND('',#3102,.T.);
#2103=FACE_OUTER_BOUND('',#3103,.T.);
#2104=FACE_OUTER_BOUND('',#3104,.T.);
#2105=FACE_OUTER_BOUND('',#3105,.T.);
#2106=FACE_OUTER_BOUND('',#3106,.T.);
#2107=FACE_OUTER_BOUND('',#3107,.T.);
#2108=FACE_OUTER_BOUND('',#3108,.T.);
#2109=FACE_OUTER_BOUND('',#3109,.T.);
#2110=FACE_OUTER_BOUND('',#3110,.T.);
#2111=FACE_OUTER_BOUND('',#3111,.T.);
#2112=FACE_OUTER_BOUND('',#3112,.T.);
#2113=FACE_OUTER_BOUND('',#3113,.T.);
#2114=FACE_OUTER_BOUND('',#3114,.T.);
#2115=FACE_OUTER_BOUND('',#3115,.T.);
#2116=FACE_OUTER_BOUND('',#3116,.T.);
#2117=FACE_OUTER_BOUND('',#3117,.T.);
#2118=FACE_OUTER_BOUND('',#3118,.T.);
#2119=FACE_OUTER_BOUND('',#3119,.T.);
#2120=FACE_OUTER_BOUND('',#3120,.T.);
#2121=FACE_OUTER_BOUND('',#3121,.T.);
#2122=FACE_OUTER_BOUND('',#3122,.T.);
#2123=FACE_OUTER_BOUND('',#3123,.T.);
#2124=FACE_OUTER_BOUND('',#3124,.T.);
#2125=FACE_OUTER_BOUND('',#3125,.T.);
#2126=FACE_OUTER_BOUND('',#3126,.T.);
#2127=FACE_OUTER_BOUND('',#3132,.T.);
#2128=FACE_OUTER_BOUND('',#3133,.T.);
#2129=FACE_OUTER_BOUND('',#3134,.T.);
#2130=FACE_OUTER_BOUND('',#3135,.T.);
#2131=FACE_OUTER_BOUND('',#3136,.T.);
#2132=FACE_OUTER_BOUND('',#3137,.T.);
#2133=FACE_OUTER_BOUND('',#3138,.T.);
#2134=FACE_OUTER_BOUND('',#3139,.T.);
#2135=FACE_OUTER_BOUND('',#3140,.T.);
#2136=FACE_OUTER_BOUND('',#3141,.T.);
#2137=FACE_OUTER_BOUND('',#3142,.T.);
#2138=FACE_OUTER_BOUND('',#3143,.T.);
#2139=FACE_OUTER_BOUND('',#3144,.T.);
#2140=FACE_OUTER_BOUND('',#3145,.T.);
#2141=FACE_OUTER_BOUND('',#3146,.T.);
#2142=FACE_OUTER_BOUND('',#3147,.T.);
#2143=FACE_OUTER_BOUND('',#3148,.T.);
#2144=FACE_OUTER_BOUND('',#3149,.T.);
#2145=FACE_OUTER_BOUND('',#3150,.T.);
#2146=FACE_OUTER_BOUND('',#3151,.T.);
#2147=FACE_OUTER_BOUND('',#3152,.T.);
#2148=FACE_OUTER_BOUND('',#3153,.T.);
#2149=FACE_OUTER_BOUND('',#3154,.T.);
#2150=FACE_OUTER_BOUND('',#3155,.T.);
#2151=FACE_OUTER_BOUND('',#3156,.T.);
#2152=FACE_OUTER_BOUND('',#3157,.T.);
#2153=FACE_OUTER_BOUND('',#3158,.T.);
#2154=FACE_OUTER_BOUND('',#3159,.T.);
#2155=FACE_OUTER_BOUND('',#3160,.T.);
#2156=FACE_OUTER_BOUND('',#3161,.T.);
#2157=FACE_OUTER_BOUND('',#3162,.T.);
#2158=FACE_OUTER_BOUND('',#3163,.T.);
#2159=FACE_OUTER_BOUND('',#3164,.T.);
#2160=FACE_OUTER_BOUND('',#3165,.T.);
#2161=FACE_OUTER_BOUND('',#3166,.T.);
#2162=FACE_OUTER_BOUND('',#3167,.T.);
#2163=FACE_OUTER_BOUND('',#3168,.T.);
#2164=FACE_OUTER_BOUND('',#3169,.T.);
#2165=FACE_OUTER_BOUND('',#3170,.T.);
#2166=FACE_OUTER_BOUND('',#3171,.T.);
#2167=FACE_OUTER_BOUND('',#3172,.T.);
#2168=FACE_OUTER_BOUND('',#3173,.T.);
#2169=FACE_OUTER_BOUND('',#3174,.T.);
#2170=FACE_OUTER_BOUND('',#3175,.T.);
#2171=FACE_OUTER_BOUND('',#3176,.T.);
#2172=FACE_OUTER_BOUND('',#3177,.T.);
#2173=FACE_OUTER_BOUND('',#3178,.T.);
#2174=FACE_OUTER_BOUND('',#3179,.T.);
#2175=FACE_OUTER_BOUND('',#3180,.T.);
#2176=FACE_OUTER_BOUND('',#3181,.T.);
#2177=FACE_OUTER_BOUND('',#3182,.T.);
#2178=FACE_OUTER_BOUND('',#3183,.T.);
#2179=FACE_OUTER_BOUND('',#3184,.T.);
#2180=FACE_OUTER_BOUND('',#3185,.T.);
#2181=FACE_OUTER_BOUND('',#3186,.T.);
#2182=FACE_OUTER_BOUND('',#3187,.T.);
#2183=FACE_OUTER_BOUND('',#3188,.T.);
#2184=FACE_OUTER_BOUND('',#3189,.T.);
#2185=FACE_OUTER_BOUND('',#3190,.T.);
#2186=FACE_OUTER_BOUND('',#3191,.T.);
#2187=FACE_OUTER_BOUND('',#3192,.T.);
#2188=FACE_OUTER_BOUND('',#3193,.T.);
#2189=FACE_OUTER_BOUND('',#3194,.T.);
#2190=FACE_OUTER_BOUND('',#3195,.T.);
#2191=FACE_OUTER_BOUND('',#3196,.T.);
#2192=FACE_OUTER_BOUND('',#3197,.T.);
#2193=FACE_OUTER_BOUND('',#3198,.T.);
#2194=FACE_OUTER_BOUND('',#3199,.T.);
#2195=FACE_OUTER_BOUND('',#3200,.T.);
#2196=FACE_OUTER_BOUND('',#3201,.T.);
#2197=FACE_OUTER_BOUND('',#3202,.T.);
#2198=FACE_OUTER_BOUND('',#3203,.T.);
#2199=FACE_OUTER_BOUND('',#3204,.T.);
#2200=FACE_OUTER_BOUND('',#3205,.T.);
#2201=FACE_OUTER_BOUND('',#3206,.T.);
#2202=FACE_OUTER_BOUND('',#3207,.T.);
#2203=FACE_OUTER_BOUND('',#3208,.T.);
#2204=FACE_OUTER_BOUND('',#3209,.T.);
#2205=FACE_OUTER_BOUND('',#3210,.T.);
#2206=FACE_OUTER_BOUND('',#3211,.T.);
#2207=FACE_OUTER_BOUND('',#3212,.T.);
#2208=FACE_OUTER_BOUND('',#3213,.T.);
#2209=FACE_OUTER_BOUND('',#3214,.T.);
#2210=FACE_OUTER_BOUND('',#3215,.T.);
#2211=FACE_OUTER_BOUND('',#3216,.T.);
#2212=FACE_OUTER_BOUND('',#3217,.T.);
#2213=FACE_OUTER_BOUND('',#3218,.T.);
#2214=FACE_OUTER_BOUND('',#3219,.T.);
#2215=FACE_OUTER_BOUND('',#3220,.T.);
#2216=FACE_OUTER_BOUND('',#3221,.T.);
#2217=FACE_OUTER_BOUND('',#3222,.T.);
#2218=FACE_OUTER_BOUND('',#3223,.T.);
#2219=FACE_OUTER_BOUND('',#3224,.T.);
#2220=FACE_OUTER_BOUND('',#3225,.T.);
#2221=FACE_OUTER_BOUND('',#3226,.T.);
#2222=FACE_OUTER_BOUND('',#3227,.T.);
#3101=EDGE_LOOP('',(#12164,#12165,#12166,#12167));
#3102=EDGE_LOOP('',(#12168,#12169,#12170,#12171,#12172,#12173));
#3103=EDGE_LOOP('',(#12174,#12175,#12176,#12177));
#3104=EDGE_LOOP('',(#12178,#12179,#12180,#12181));
#3105=EDGE_LOOP('',(#12182,#12183,#12184,#12185));
#3106=EDGE_LOOP('',(#12186,#12187,#12188,#12189,#12190,#12191));
#3107=EDGE_LOOP('',(#12192,#12193,#12194,#12195,#12196,#12197));
#3108=EDGE_LOOP('',(#12198,#12199,#12200,#12201));
#3109=EDGE_LOOP('',(#12202,#12203,#12204,#12205,#12206,#12207));
#3110=EDGE_LOOP('',(#12208,#12209,#12210,#12211,#12212));
#3111=EDGE_LOOP('',(#12213,#12214,#12215,#12216,#12217));
#3112=EDGE_LOOP('',(#12218,#12219,#12220,#12221));
#3113=EDGE_LOOP('',(#12222,#12223,#12224,#12225,#12226));
#3114=EDGE_LOOP('',(#12227,#12228,#12229,#12230,#12231,#12232));
#3115=EDGE_LOOP('',(#12233,#12234,#12235,#12236,#12237,#12238,#12239,#12240));
#3116=EDGE_LOOP('',(#12241,#12242,#12243,#12244,#12245,#12246));
#3117=EDGE_LOOP('',(#12247,#12248,#12249,#12250));
#3118=EDGE_LOOP('',(#12251,#12252,#12253,#12254,#12255,#12256));
#3119=EDGE_LOOP('',(#12257,#12258,#12259,#12260));
#3120=EDGE_LOOP('',(#12261,#12262,#12263,#12264));
#3121=EDGE_LOOP('',(#12265,#12266,#12267,#12268));
#3122=EDGE_LOOP('',(#12269,#12270,#12271,#12272,#12273,#12274));
#3123=EDGE_LOOP('',(#12275,#12276,#12277,#12278));
#3124=EDGE_LOOP('',(#12279,#12280,#12281,#12282,#12283));
#3125=EDGE_LOOP('',(#12284,#12285,#12286,#12287));
#3126=EDGE_LOOP('',(#12288,#12289,#12290,#12291,#12292,#12293,#12294,#12295));
#3127=EDGE_LOOP('',(#12296,#12297,#12298,#12299,#12300,#12301,#12302,#12303,
#12304,#12305,#12306,#12307,#12308,#12309,#12310,#12311,#12312,#12313,#12314));
#3128=EDGE_LOOP('',(#12315,#12316,#12317,#12318,#12319,#12320,#12321,#12322));
#3129=EDGE_LOOP('',(#12323,#12324,#12325,#12326,#12327,#12328,#12329,#12330,
#12331,#12332,#12333,#12334));
#3130=EDGE_LOOP('',(#12335,#12336,#12337,#12338,#12339,#12340,#12341,#12342,
#12343));
#3131=EDGE_LOOP('',(#12344,#12345,#12346,#12347,#12348,#12349,#12350,#12351,
#12352,#12353,#12354,#12355,#12356,#12357,#12358,#12359,#12360,#12361,#12362,
#12363,#12364,#12365,#12366,#12367,#12368,#12369,#12370,#12371,#12372));
#3132=EDGE_LOOP('',(#12373,#12374,#12375,#12376,#12377,#12378));
#3133=EDGE_LOOP('',(#12379,#12380,#12381,#12382,#12383,#12384));
#3134=EDGE_LOOP('',(#12385,#12386,#12387,#12388));
#3135=EDGE_LOOP('',(#12389,#12390,#12391,#12392));
#3136=EDGE_LOOP('',(#12393,#12394,#12395,#12396,#12397,#12398));
#3137=EDGE_LOOP('',(#12399,#12400,#12401,#12402,#12403,#12404));
#3138=EDGE_LOOP('',(#12405,#12406,#12407,#12408));
#3139=EDGE_LOOP('',(#12409,#12410,#12411,#12412));
#3140=EDGE_LOOP('',(#12413,#12414,#12415,#12416));
#3141=EDGE_LOOP('',(#12417,#12418,#12419,#12420));
#3142=EDGE_LOOP('',(#12421,#12422,#12423,#12424));
#3143=EDGE_LOOP('',(#12425,#12426,#12427,#12428));
#3144=EDGE_LOOP('',(#12429,#12430,#12431,#12432));
#3145=EDGE_LOOP('',(#12433,#12434,#12435,#12436));
#3146=EDGE_LOOP('',(#12437,#12438,#12439,#12440));
#3147=EDGE_LOOP('',(#12441,#12442,#12443,#12444));
#3148=EDGE_LOOP('',(#12445,#12446,#12447,#12448));
#3149=EDGE_LOOP('',(#12449,#12450,#12451,#12452));
#3150=EDGE_LOOP('',(#12453,#12454,#12455,#12456));
#3151=EDGE_LOOP('',(#12457,#12458,#12459,#12460));
#3152=EDGE_LOOP('',(#12461,#12462,#12463,#12464));
#3153=EDGE_LOOP('',(#12465,#12466,#12467,#12468));
#3154=EDGE_LOOP('',(#12469,#12470,#12471,#12472));
#3155=EDGE_LOOP('',(#12473,#12474,#12475,#12476));
#3156=EDGE_LOOP('',(#12477,#12478,#12479,#12480));
#3157=EDGE_LOOP('',(#12481,#12482,#12483,#12484));
#3158=EDGE_LOOP('',(#12485,#12486,#12487,#12488,#12489,#12490,#12491,#12492,
#12493,#12494,#12495,#12496,#12497,#12498,#12499,#12500,#12501,#12502,#12503));
#3159=EDGE_LOOP('',(#12504,#12505,#12506,#12507));
#3160=EDGE_LOOP('',(#12508,#12509,#12510,#12511));
#3161=EDGE_LOOP('',(#12512,#12513,#12514,#12515));
#3162=EDGE_LOOP('',(#12516,#12517,#12518,#12519));
#3163=EDGE_LOOP('',(#12520,#12521,#12522,#12523));
#3164=EDGE_LOOP('',(#12524,#12525,#12526,#12527));
#3165=EDGE_LOOP('',(#12528,#12529,#12530,#12531));
#3166=EDGE_LOOP('',(#12532,#12533,#12534,#12535));
#3167=EDGE_LOOP('',(#12536,#12537,#12538,#12539,#12540,#12541,#12542,#12543));
#3168=EDGE_LOOP('',(#12544,#12545,#12546,#12547));
#3169=EDGE_LOOP('',(#12548,#12549,#12550,#12551));
#3170=EDGE_LOOP('',(#12552,#12553,#12554,#12555));
#3171=EDGE_LOOP('',(#12556,#12557,#12558,#12559));
#3172=EDGE_LOOP('',(#12560,#12561,#12562,#12563));
#3173=EDGE_LOOP('',(#12564,#12565,#12566,#12567));
#3174=EDGE_LOOP('',(#12568,#12569,#12570,#12571));
#3175=EDGE_LOOP('',(#12572,#12573,#12574,#12575));
#3176=EDGE_LOOP('',(#12576,#12577,#12578,#12579));
#3177=EDGE_LOOP('',(#12580,#12581,#12582,#12583));
#3178=EDGE_LOOP('',(#12584,#12585,#12586,#12587));
#3179=EDGE_LOOP('',(#12588,#12589,#12590,#12591));
#3180=EDGE_LOOP('',(#12592,#12593,#12594,#12595,#12596,#12597,#12598,#12599,
#12600,#12601,#12602,#12603));
#3181=EDGE_LOOP('',(#12604,#12605,#12606,#12607));
#3182=EDGE_LOOP('',(#12608,#12609,#12610,#12611));
#3183=EDGE_LOOP('',(#12612,#12613,#12614,#12615));
#3184=EDGE_LOOP('',(#12616,#12617,#12618,#12619));
#3185=EDGE_LOOP('',(#12620,#12621,#12622,#12623));
#3186=EDGE_LOOP('',(#12624,#12625,#12626,#12627));
#3187=EDGE_LOOP('',(#12628,#12629,#12630,#12631));
#3188=EDGE_LOOP('',(#12632,#12633,#12634,#12635));
#3189=EDGE_LOOP('',(#12636,#12637,#12638,#12639));
#3190=EDGE_LOOP('',(#12640,#12641,#12642,#12643,#12644,#12645,#12646,#12647,
#12648));
#3191=EDGE_LOOP('',(#12649,#12650,#12651,#12652));
#3192=EDGE_LOOP('',(#12653,#12654,#12655,#12656));
#3193=EDGE_LOOP('',(#12657,#12658,#12659,#12660));
#3194=EDGE_LOOP('',(#12661,#12662,#12663,#12664));
#3195=EDGE_LOOP('',(#12665,#12666,#12667,#12668));
#3196=EDGE_LOOP('',(#12669,#12670,#12671,#12672));
#3197=EDGE_LOOP('',(#12673,#12674,#12675,#12676));
#3198=EDGE_LOOP('',(#12677,#12678,#12679,#12680));
#3199=EDGE_LOOP('',(#12681,#12682,#12683,#12684));
#3200=EDGE_LOOP('',(#12685,#12686,#12687,#12688));
#3201=EDGE_LOOP('',(#12689,#12690,#12691,#12692));
#3202=EDGE_LOOP('',(#12693,#12694,#12695,#12696));
#3203=EDGE_LOOP('',(#12697,#12698,#12699,#12700));
#3204=EDGE_LOOP('',(#12701,#12702,#12703,#12704));
#3205=EDGE_LOOP('',(#12705,#12706,#12707,#12708));
#3206=EDGE_LOOP('',(#12709,#12710,#12711,#12712));
#3207=EDGE_LOOP('',(#12713,#12714,#12715,#12716));
#3208=EDGE_LOOP('',(#12717,#12718,#12719,#12720));
#3209=EDGE_LOOP('',(#12721,#12722,#12723,#12724));
#3210=EDGE_LOOP('',(#12725,#12726,#12727,#12728));
#3211=EDGE_LOOP('',(#12729,#12730,#12731,#12732));
#3212=EDGE_LOOP('',(#12733,#12734,#12735,#12736));
#3213=EDGE_LOOP('',(#12737,#12738,#12739,#12740));
#3214=EDGE_LOOP('',(#12741,#12742,#12743,#12744));
#3215=EDGE_LOOP('',(#12745,#12746,#12747,#12748));
#3216=EDGE_LOOP('',(#12749,#12750,#12751,#12752));
#3217=EDGE_LOOP('',(#12753,#12754,#12755,#12756));
#3218=EDGE_LOOP('',(#12757,#12758,#12759,#12760));
#3219=EDGE_LOOP('',(#12761,#12762,#12763,#12764));
#3220=EDGE_LOOP('',(#12765,#12766,#12767,#12768,#12769,#12770,#12771,#12772,
#12773,#12774,#12775,#12776,#12777,#12778,#12779,#12780,#12781,#12782,#12783,
#12784,#12785,#12786,#12787,#12788,#12789,#12790,#12791,#12792,#12793));
#3221=EDGE_LOOP('',(#12794,#12795,#12796,#12797,#12798,#12799));
#3222=EDGE_LOOP('',(#12800,#12801,#12802,#12803,#12804,#12805));
#3223=EDGE_LOOP('',(#12806,#12807,#12808,#12809,#12810,#12811));
#3224=EDGE_LOOP('',(#12812,#12813,#12814,#12815));
#3225=EDGE_LOOP('',(#12816,#12817,#12818,#12819,#12820,#12821));
#3226=EDGE_LOOP('',(#12822,#12823,#12824,#12825));
#3227=EDGE_LOOP('',(#12826,#12827,#12828,#12829));
#4171=LINE('',#32268,#5482);
#4172=LINE('',#32270,#5483);
#4173=LINE('',#32272,#5484);
#4174=LINE('',#32273,#5485);
#4175=LINE('',#32276,#5486);
#4176=LINE('',#32278,#5487);
#4177=LINE('',#32280,#5488);
#4178=LINE('',#32282,#5489);
#4179=LINE('',#32283,#5490);
#4180=LINE('',#32286,#5491);
#4181=LINE('',#32287,#5492);
#4182=LINE('',#32291,#5493);
#4183=LINE('',#32293,#5494);
#4184=LINE('',#32295,#5495);
#4185=LINE('',#32296,#5496);
#4186=LINE('',#32299,#5497);
#4187=LINE('',#32301,#5498);
#4188=LINE('',#32302,#5499);
#4189=LINE('',#32304,#5500);
#4190=LINE('',#32306,#5501);
#4191=LINE('',#32308,#5502);
#4192=LINE('',#32309,#5503);
#4193=LINE('',#32313,#5504);
#4194=LINE('',#32315,#5505);
#4195=LINE('',#32317,#5506);
#4196=LINE('',#32319,#5507);
#4197=LINE('',#32321,#5508);
#4198=LINE('',#32322,#5509);
#4199=LINE('',#32325,#5510);
#4200=LINE('',#32327,#5511);
#4201=LINE('',#32328,#5512);
#4202=LINE('',#32331,#5513);
#4203=LINE('',#32333,#5514);
#4204=LINE('',#32335,#5515);
#4205=LINE('',#32336,#5516);
#4206=LINE('',#32339,#5517);
#4207=LINE('',#32341,#5518);
#4208=LINE('',#32342,#5519);
#4209=LINE('',#32346,#5520);
#4210=LINE('',#32348,#5521);
#4211=LINE('',#32350,#5522);
#4212=LINE('',#32352,#5523);
#4213=LINE('',#32353,#5524);
#4214=LINE('',#32356,#5525);
#4215=LINE('',#32358,#5526);
#4216=LINE('',#32359,#5527);
#4217=LINE('',#32362,#5528);
#4218=LINE('',#32363,#5529);
#4219=LINE('',#32364,#5530);
#4220=LINE('',#32367,#5531);
#4221=LINE('',#32369,#5532);
#4222=LINE('',#32371,#5533);
#4223=LINE('',#32373,#5534);
#4224=LINE('',#32374,#5535);
#4225=LINE('',#32377,#5536);
#4226=LINE('',#32379,#5537);
#4227=LINE('',#32381,#5538);
#4228=LINE('',#32382,#5539);
#4229=LINE('',#32385,#5540);
#4230=LINE('',#32386,#5541);
#4231=LINE('',#32390,#5542);
#4232=LINE('',#32392,#5543);
#4233=LINE('',#32394,#5544);
#4234=LINE('',#32395,#5545);
#4235=LINE('',#32398,#5546);
#4236=LINE('',#32400,#5547);
#4237=LINE('',#32401,#5548);
#4238=LINE('',#32402,#5549);
#4239=LINE('',#32403,#5550);
#4240=LINE('',#32406,#5551);
#4241=LINE('',#32407,#5552);
#4242=LINE('',#32410,#5553);
#4243=LINE('',#32411,#5554);
#4244=LINE('',#32413,#5555);
#4245=LINE('',#32416,#5556);
#4246=LINE('',#32417,#5557);
#4247=LINE('',#32419,#5558);
#4248=LINE('',#32423,#5559);
#4249=LINE('',#32425,#5560);
#4250=LINE('',#32427,#5561);
#4251=LINE('',#32429,#5562);
#4252=LINE('',#32430,#5563);
#4253=LINE('',#32432,#5564);
#4254=LINE('',#32433,#5565);
#4255=LINE('',#32435,#5566);
#4256=LINE('',#32442,#5567);
#4257=LINE('',#32444,#5568);
#4258=LINE('',#32446,#5569);
#4259=LINE('',#32448,#5570);
#4260=LINE('',#32450,#5571);
#4261=LINE('',#32460,#5572);
#4262=LINE('',#32462,#5573);
#4263=LINE('',#32464,#5574);
#4264=LINE('',#32474,#5575);
#4265=LINE('',#32476,#5576);
#4266=LINE('',#32478,#5577);
#4267=LINE('',#32480,#5578);
#4268=LINE('',#32482,#5579);
#4269=LINE('',#32488,#5580);
#4270=LINE('',#32490,#5581);
#4271=LINE('',#32492,#5582);
#4272=LINE('',#32494,#5583);
#4273=LINE('',#32496,#5584);
#4274=LINE('',#32498,#5585);
#4275=LINE('',#32500,#5586);
#4276=LINE('',#32501,#5587);
#4277=LINE('',#32556,#5588);
#4278=LINE('',#32558,#5589);
#4279=LINE('',#32560,#5590);
#4280=LINE('',#32562,#5591);
#4281=LINE('',#32572,#5592);
#4282=LINE('',#32582,#5593);
#4283=LINE('',#32584,#5594);
#4284=LINE('',#32586,#5595);
#4285=LINE('',#32588,#5596);
#4286=LINE('',#32590,#5597);
#4287=LINE('',#32636,#5598);
#4288=LINE('',#32682,#5599);
#4289=LINE('',#32684,#5600);
#4290=LINE('',#32686,#5601);
#4291=LINE('',#32687,#5602);
#4292=LINE('',#32689,#5603);
#4293=LINE('',#32690,#5604);
#4294=LINE('',#32692,#5605);
#4295=LINE('',#32695,#5606);
#4296=LINE('',#32696,#5607);
#4297=LINE('',#32698,#5608);
#4298=LINE('',#32699,#5609);
#4299=LINE('',#32701,#5610);
#4300=LINE('',#32710,#5611);
#4301=LINE('',#32715,#5612);
#4302=LINE('',#32723,#5613);
#4303=LINE('',#32729,#5614);
#4304=LINE('',#32730,#5615);
#4305=LINE('',#32733,#5616);
#4306=LINE('',#32734,#5617);
#4307=LINE('',#32737,#5618);
#4308=LINE('',#32738,#5619);
#4309=LINE('',#32741,#5620);
#4310=LINE('',#32742,#5621);
#4311=LINE('',#32745,#5622);
#4312=LINE('',#32746,#5623);
#4313=LINE('',#32754,#5624);
#4314=LINE('',#32765,#5625);
#4315=LINE('',#32771,#5626);
#4316=LINE('',#32772,#5627);
#4317=LINE('',#32775,#5628);
#4318=LINE('',#32776,#5629);
#4319=LINE('',#32779,#5630);
#4320=LINE('',#32780,#5631);
#4321=LINE('',#32788,#5632);
#4322=LINE('',#32799,#5633);
#4323=LINE('',#32805,#5634);
#4324=LINE('',#32806,#5635);
#4325=LINE('',#32809,#5636);
#4326=LINE('',#32810,#5637);
#4327=LINE('',#32813,#5638);
#4328=LINE('',#32814,#5639);
#4329=LINE('',#32817,#5640);
#4330=LINE('',#32818,#5641);
#4331=LINE('',#32820,#5642);
#4332=LINE('',#32824,#5643);
#4333=LINE('',#32826,#5644);
#4334=LINE('',#32827,#5645);
#4335=LINE('',#32830,#5646);
#4336=LINE('',#32831,#5647);
#4337=LINE('',#32834,#5648);
#4338=LINE('',#32835,#5649);
#4339=LINE('',#32838,#5650);
#4340=LINE('',#32839,#5651);
#4341=LINE('',#32842,#5652);
#4342=LINE('',#32843,#5653);
#4343=LINE('',#32846,#5654);
#4344=LINE('',#32847,#5655);
#4345=LINE('',#32850,#5656);
#4346=LINE('',#32851,#5657);
#4347=LINE('',#32853,#5658);
#4348=LINE('',#32862,#5659);
#4349=LINE('',#32867,#5660);
#4350=LINE('',#32875,#5661);
#4351=LINE('',#32886,#5662);
#4352=LINE('',#32897,#5663);
#4353=LINE('',#32908,#5664);
#4354=LINE('',#32919,#5665);
#4355=LINE('',#32930,#5666);
#4356=LINE('',#32941,#5667);
#4357=LINE('',#32952,#5668);
#4358=LINE('',#32963,#5669);
#4359=LINE('',#32974,#5670);
#4360=LINE('',#32995,#5671);
#4361=LINE('',#33000,#5672);
#4362=LINE('',#33008,#5673);
#4363=LINE('',#33014,#5674);
#4364=LINE('',#33015,#5675);
#4365=LINE('',#33023,#5676);
#4366=LINE('',#33034,#5677);
#4367=LINE('',#33040,#5678);
#4368=LINE('',#33041,#5679);
#4369=LINE('',#33044,#5680);
#4370=LINE('',#33045,#5681);
#4371=LINE('',#33048,#5682);
#4372=LINE('',#33049,#5683);
#4373=LINE('',#33051,#5684);
#4374=LINE('',#33060,#5685);
#4375=LINE('',#33065,#5686);
#4376=LINE('',#33073,#5687);
#4377=LINE('',#33084,#5688);
#4378=LINE('',#33095,#5689);
#4379=LINE('',#33106,#5690);
#4380=LINE('',#33117,#5691);
#4381=LINE('',#33128,#5692);
#4382=LINE('',#33139,#5693);
#4383=LINE('',#33150,#5694);
#4384=LINE('',#33161,#5695);
#4385=LINE('',#33172,#5696);
#4386=LINE('',#33183,#5697);
#4387=LINE('',#33189,#5698);
#4388=LINE('',#33190,#5699);
#4389=LINE('',#33198,#5700);
#4390=LINE('',#33209,#5701);
#4391=LINE('',#33220,#5702);
#4392=LINE('',#33231,#5703);
#4393=LINE('',#33242,#5704);
#4394=LINE('',#33253,#5705);
#4395=LINE('',#33264,#5706);
#4396=LINE('',#33275,#5707);
#4397=LINE('',#33286,#5708);
#4398=LINE('',#33297,#5709);
#4399=LINE('',#33308,#5710);
#4400=LINE('',#33314,#5711);
#4401=LINE('',#33315,#5712);
#4402=LINE('',#33318,#5713);
#4403=LINE('',#33319,#5714);
#4404=LINE('',#33322,#5715);
#4405=LINE('',#33323,#5716);
#4406=LINE('',#33326,#5717);
#4407=LINE('',#33327,#5718);
#4408=LINE('',#33329,#5719);
#4409=LINE('',#33332,#5720);
#4410=LINE('',#33333,#5721);
#4411=LINE('',#33335,#5722);
#4412=LINE('',#33338,#5723);
#4413=LINE('',#33341,#5724);
#5482=VECTOR('',#19246,10.);
#5483=VECTOR('',#19247,10.);
#5484=VECTOR('',#19248,10.);
#5485=VECTOR('',#19249,10.);
#5486=VECTOR('',#19252,10.);
#5487=VECTOR('',#19253,10.);
#5488=VECTOR('',#19254,10.);
#5489=VECTOR('',#19255,10.);
#5490=VECTOR('',#19256,10.);
#5491=VECTOR('',#19259,10.);
#5492=VECTOR('',#19260,10.);
#5493=VECTOR('',#19263,10.);
#5494=VECTOR('',#19264,10.);
#5495=VECTOR('',#19265,10.);
#5496=VECTOR('',#19266,10.);
#5497=VECTOR('',#19269,10.);
#5498=VECTOR('',#19270,10.);
#5499=VECTOR('',#19271,10.);
#5500=VECTOR('',#19274,10.);
#5501=VECTOR('',#19275,10.);
#5502=VECTOR('',#19276,10.);
#5503=VECTOR('',#19277,10.);
#5504=VECTOR('',#19280,10.);
#5505=VECTOR('',#19281,10.);
#5506=VECTOR('',#19282,10.);
#5507=VECTOR('',#19283,10.);
#5508=VECTOR('',#19284,10.);
#5509=VECTOR('',#19285,10.);
#5510=VECTOR('',#19288,10.);
#5511=VECTOR('',#19289,10.);
#5512=VECTOR('',#19290,10.);
#5513=VECTOR('',#19293,10.);
#5514=VECTOR('',#19294,10.);
#5515=VECTOR('',#19295,10.);
#5516=VECTOR('',#19296,10.);
#5517=VECTOR('',#19299,10.);
#5518=VECTOR('',#19300,10.);
#5519=VECTOR('',#19301,10.);
#5520=VECTOR('',#19304,10.);
#5521=VECTOR('',#19305,10.);
#5522=VECTOR('',#19306,10.);
#5523=VECTOR('',#19307,10.);
#5524=VECTOR('',#19308,10.);
#5525=VECTOR('',#19311,10.);
#5526=VECTOR('',#19312,10.);
#5527=VECTOR('',#19313,10.);
#5528=VECTOR('',#19316,10.);
#5529=VECTOR('',#19317,10.);
#5530=VECTOR('',#19318,10.);
#5531=VECTOR('',#19321,10.);
#5532=VECTOR('',#19322,10.);
#5533=VECTOR('',#19323,10.);
#5534=VECTOR('',#19324,10.);
#5535=VECTOR('',#19325,10.);
#5536=VECTOR('',#19328,10.);
#5537=VECTOR('',#19329,10.);
#5538=VECTOR('',#19330,10.);
#5539=VECTOR('',#19331,10.);
#5540=VECTOR('',#19334,10.);
#5541=VECTOR('',#19335,10.);
#5542=VECTOR('',#19338,10.);
#5543=VECTOR('',#19339,10.);
#5544=VECTOR('',#19340,10.);
#5545=VECTOR('',#19341,10.);
#5546=VECTOR('',#19344,10.);
#5547=VECTOR('',#19345,10.);
#5548=VECTOR('',#19346,10.);
#5549=VECTOR('',#19347,10.);
#5550=VECTOR('',#19348,10.);
#5551=VECTOR('',#19351,10.);
#5552=VECTOR('',#19352,10.);
#5553=VECTOR('',#19355,10.);
#5554=VECTOR('',#19356,10.);
#5555=VECTOR('',#19359,10.);
#5556=VECTOR('',#19362,10.);
#5557=VECTOR('',#19363,10.);
#5558=VECTOR('',#19366,10.);
#5559=VECTOR('',#19369,10.);
#5560=VECTOR('',#19370,10.);
#5561=VECTOR('',#19371,10.);
#5562=VECTOR('',#19372,10.);
#5563=VECTOR('',#19373,10.);
#5564=VECTOR('',#19376,10.);
#5565=VECTOR('',#19377,10.);
#5566=VECTOR('',#19380,10.);
#5567=VECTOR('',#19381,10.);
#5568=VECTOR('',#19382,10.);
#5569=VECTOR('',#19383,10.);
#5570=VECTOR('',#19384,10.);
#5571=VECTOR('',#19385,10.);
#5572=VECTOR('',#19386,10.);
#5573=VECTOR('',#19387,10.);
#5574=VECTOR('',#19388,10.);
#5575=VECTOR('',#19389,10.);
#5576=VECTOR('',#19390,10.);
#5577=VECTOR('',#19391,10.);
#5578=VECTOR('',#19392,10.);
#5579=VECTOR('',#19393,10.);
#5580=VECTOR('',#19394,10.);
#5581=VECTOR('',#19395,10.);
#5582=VECTOR('',#19396,10.);
#5583=VECTOR('',#19397,10.);
#5584=VECTOR('',#19398,10.);
#5585=VECTOR('',#19399,10.);
#5586=VECTOR('',#19400,10.);
#5587=VECTOR('',#19401,10.);
#5588=VECTOR('',#19402,10.);
#5589=VECTOR('',#19403,10.);
#5590=VECTOR('',#19404,10.);
#5591=VECTOR('',#19405,10.);
#5592=VECTOR('',#19406,10.);
#5593=VECTOR('',#19407,10.);
#5594=VECTOR('',#19408,10.);
#5595=VECTOR('',#19409,10.);
#5596=VECTOR('',#19410,10.);
#5597=VECTOR('',#19411,10.);
#5598=VECTOR('',#19412,10.);
#5599=VECTOR('',#19415,10.);
#5600=VECTOR('',#19416,10.);
#5601=VECTOR('',#19417,10.);
#5602=VECTOR('',#19418,10.);
#5603=VECTOR('',#19421,10.);
#5604=VECTOR('',#19422,10.);
#5605=VECTOR('',#19425,10.);
#5606=VECTOR('',#19428,10.);
#5607=VECTOR('',#19429,10.);
#5608=VECTOR('',#19432,10.);
#5609=VECTOR('',#19433,10.);
#5610=VECTOR('',#19436,10.);
#5611=VECTOR('',#19439,10.);
#5612=VECTOR('',#19440,10.);
#5613=VECTOR('',#19441,10.);
#5614=VECTOR('',#19444,10.);
#5615=VECTOR('',#19445,10.);
#5616=VECTOR('',#19448,10.);
#5617=VECTOR('',#19449,10.);
#5618=VECTOR('',#19452,10.);
#5619=VECTOR('',#19453,10.);
#5620=VECTOR('',#19456,10.);
#5621=VECTOR('',#19457,10.);
#5622=VECTOR('',#19460,10.);
#5623=VECTOR('',#19461,10.);
#5624=VECTOR('',#19462,10.);
#5625=VECTOR('',#19463,10.);
#5626=VECTOR('',#19466,10.);
#5627=VECTOR('',#19467,10.);
#5628=VECTOR('',#19470,10.);
#5629=VECTOR('',#19471,10.);
#5630=VECTOR('',#19474,10.);
#5631=VECTOR('',#19475,10.);
#5632=VECTOR('',#19476,10.);
#5633=VECTOR('',#19477,10.);
#5634=VECTOR('',#19480,10.);
#5635=VECTOR('',#19481,10.);
#5636=VECTOR('',#19484,10.);
#5637=VECTOR('',#19485,10.);
#5638=VECTOR('',#19488,10.);
#5639=VECTOR('',#19489,10.);
#5640=VECTOR('',#19492,10.);
#5641=VECTOR('',#19493,10.);
#5642=VECTOR('',#19496,10.);
#5643=VECTOR('',#19501,10.);
#5644=VECTOR('',#19502,10.);
#5645=VECTOR('',#19503,10.);
#5646=VECTOR('',#19506,10.);
#5647=VECTOR('',#19507,10.);
#5648=VECTOR('',#19510,10.);
#5649=VECTOR('',#19511,10.);
#5650=VECTOR('',#19514,10.);
#5651=VECTOR('',#19515,10.);
#5652=VECTOR('',#19518,10.);
#5653=VECTOR('',#19519,10.);
#5654=VECTOR('',#19522,10.);
#5655=VECTOR('',#19523,10.);
#5656=VECTOR('',#19526,10.);
#5657=VECTOR('',#19527,10.);
#5658=VECTOR('',#19530,10.);
#5659=VECTOR('',#19533,10.);
#5660=VECTOR('',#19534,10.);
#5661=VECTOR('',#19535,10.);
#5662=VECTOR('',#19536,10.);
#5663=VECTOR('',#19537,10.);
#5664=VECTOR('',#19538,10.);
#5665=VECTOR('',#19539,10.);
#5666=VECTOR('',#19540,10.);
#5667=VECTOR('',#19541,10.);
#5668=VECTOR('',#19542,10.);
#5669=VECTOR('',#19543,10.);
#5670=VECTOR('',#19544,10.);
#5671=VECTOR('',#19547,10.);
#5672=VECTOR('',#19548,10.);
#5673=VECTOR('',#19549,10.);
#5674=VECTOR('',#19552,10.);
#5675=VECTOR('',#19553,10.);
#5676=VECTOR('',#19554,10.);
#5677=VECTOR('',#19555,10.);
#5678=VECTOR('',#19558,10.);
#5679=VECTOR('',#19559,10.);
#5680=VECTOR('',#19562,10.);
#5681=VECTOR('',#19563,10.);
#5682=VECTOR('',#19566,10.);
#5683=VECTOR('',#19567,10.);
#5684=VECTOR('',#19570,10.);
#5685=VECTOR('',#19573,10.);
#5686=VECTOR('',#19574,10.);
#5687=VECTOR('',#19575,10.);
#5688=VECTOR('',#19576,10.);
#5689=VECTOR('',#19577,10.);
#5690=VECTOR('',#19578,10.);
#5691=VECTOR('',#19579,10.);
#5692=VECTOR('',#19580,10.);
#5693=VECTOR('',#19581,10.);
#5694=VECTOR('',#19582,10.);
#5695=VECTOR('',#19583,10.);
#5696=VECTOR('',#19584,10.);
#5697=VECTOR('',#19585,10.);
#5698=VECTOR('',#19588,10.);
#5699=VECTOR('',#19589,10.);
#5700=VECTOR('',#19590,10.);
#5701=VECTOR('',#19591,10.);
#5702=VECTOR('',#19592,10.);
#5703=VECTOR('',#19593,10.);
#5704=VECTOR('',#19594,10.);
#5705=VECTOR('',#19595,10.);
#5706=VECTOR('',#19596,10.);
#5707=VECTOR('',#19597,10.);
#5708=VECTOR('',#19598,10.);
#5709=VECTOR('',#19599,10.);
#5710=VECTOR('',#19600,10.);
#5711=VECTOR('',#19603,10.);
#5712=VECTOR('',#19604,10.);
#5713=VECTOR('',#19607,10.);
#5714=VECTOR('',#19608,10.);
#5715=VECTOR('',#19611,10.);
#5716=VECTOR('',#19612,10.);
#5717=VECTOR('',#19615,10.);
#5718=VECTOR('',#19616,10.);
#5719=VECTOR('',#19619,10.);
#5720=VECTOR('',#19624,10.);
#5721=VECTOR('',#19625,10.);
#5722=VECTOR('',#19628,10.);
#5723=VECTOR('',#19633,10.);
#5724=VECTOR('',#19638,10.);
#7388=VERTEX_POINT('',#32266);
#7389=VERTEX_POINT('',#32267);
#7390=VERTEX_POINT('',#32269);
#7391=VERTEX_POINT('',#32271);
#7392=VERTEX_POINT('',#32275);
#7393=VERTEX_POINT('',#32277);
#7394=VERTEX_POINT('',#32279);
#7395=VERTEX_POINT('',#32281);
#7396=VERTEX_POINT('',#32285);
#7397=VERTEX_POINT('',#32289);
#7398=VERTEX_POINT('',#32290);
#7399=VERTEX_POINT('',#32292);
#7400=VERTEX_POINT('',#32294);
#7401=VERTEX_POINT('',#32298);
#7402=VERTEX_POINT('',#32300);
#7403=VERTEX_POINT('',#32305);
#7404=VERTEX_POINT('',#32307);
#7405=VERTEX_POINT('',#32311);
#7406=VERTEX_POINT('',#32312);
#7407=VERTEX_POINT('',#32314);
#7408=VERTEX_POINT('',#32316);
#7409=VERTEX_POINT('',#32318);
#7410=VERTEX_POINT('',#32320);
#7411=VERTEX_POINT('',#32324);
#7412=VERTEX_POINT('',#32326);
#7413=VERTEX_POINT('',#32330);
#7414=VERTEX_POINT('',#32332);
#7415=VERTEX_POINT('',#32334);
#7416=VERTEX_POINT('',#32338);
#7417=VERTEX_POINT('',#32340);
#7418=VERTEX_POINT('',#32344);
#7419=VERTEX_POINT('',#32345);
#7420=VERTEX_POINT('',#32347);
#7421=VERTEX_POINT('',#32349);
#7422=VERTEX_POINT('',#32351);
#7423=VERTEX_POINT('',#32355);
#7424=VERTEX_POINT('',#32357);
#7425=VERTEX_POINT('',#32361);
#7426=VERTEX_POINT('',#32366);
#7427=VERTEX_POINT('',#32368);
#7428=VERTEX_POINT('',#32370);
#7429=VERTEX_POINT('',#32372);
#7430=VERTEX_POINT('',#32376);
#7431=VERTEX_POINT('',#32378);
#7432=VERTEX_POINT('',#32380);
#7433=VERTEX_POINT('',#32384);
#7434=VERTEX_POINT('',#32388);
#7435=VERTEX_POINT('',#32389);
#7436=VERTEX_POINT('',#32391);
#7437=VERTEX_POINT('',#32393);
#7438=VERTEX_POINT('',#32397);
#7439=VERTEX_POINT('',#32399);
#7440=VERTEX_POINT('',#32405);
#7441=VERTEX_POINT('',#32409);
#7442=VERTEX_POINT('',#32415);
#7443=VERTEX_POINT('',#32421);
#7444=VERTEX_POINT('',#32422);
#7445=VERTEX_POINT('',#32424);
#7446=VERTEX_POINT('',#32426);
#7447=VERTEX_POINT('',#32428);
#7448=VERTEX_POINT('',#32436);
#7449=VERTEX_POINT('',#32437);
#7450=VERTEX_POINT('',#32441);
#7451=VERTEX_POINT('',#32443);
#7452=VERTEX_POINT('',#32445);
#7453=VERTEX_POINT('',#32447);
#7454=VERTEX_POINT('',#32449);
#7455=VERTEX_POINT('',#32451);
#7456=VERTEX_POINT('',#32455);
#7457=VERTEX_POINT('',#32459);
#7458=VERTEX_POINT('',#32461);
#7459=VERTEX_POINT('',#32463);
#7460=VERTEX_POINT('',#32465);
#7461=VERTEX_POINT('',#32469);
#7462=VERTEX_POINT('',#32473);
#7463=VERTEX_POINT('',#32475);
#7464=VERTEX_POINT('',#32477);
#7465=VERTEX_POINT('',#32479);
#7466=VERTEX_POINT('',#32481);
#7467=VERTEX_POINT('',#32486);
#7468=VERTEX_POINT('',#32487);
#7469=VERTEX_POINT('',#32489);
#7470=VERTEX_POINT('',#32491);
#7471=VERTEX_POINT('',#32493);
#7472=VERTEX_POINT('',#32495);
#7473=VERTEX_POINT('',#32497);
#7474=VERTEX_POINT('',#32499);
#7475=VERTEX_POINT('',#32502);
#7476=VERTEX_POINT('',#32503);
#7477=VERTEX_POINT('',#32507);
#7478=VERTEX_POINT('',#32511);
#7479=VERTEX_POINT('',#32515);
#7480=VERTEX_POINT('',#32519);
#7481=VERTEX_POINT('',#32523);
#7482=VERTEX_POINT('',#32527);
#7483=VERTEX_POINT('',#32531);
#7484=VERTEX_POINT('',#32535);
#7485=VERTEX_POINT('',#32539);
#7486=VERTEX_POINT('',#32543);
#7487=VERTEX_POINT('',#32550);
#7488=VERTEX_POINT('',#32551);
#7489=VERTEX_POINT('',#32555);
#7490=VERTEX_POINT('',#32557);
#7491=VERTEX_POINT('',#32559);
#7492=VERTEX_POINT('',#32561);
#7493=VERTEX_POINT('',#32563);
#7494=VERTEX_POINT('',#32567);
#7495=VERTEX_POINT('',#32571);
#7496=VERTEX_POINT('',#32576);
#7497=VERTEX_POINT('',#32577);
#7498=VERTEX_POINT('',#32581);
#7499=VERTEX_POINT('',#32583);
#7500=VERTEX_POINT('',#32585);
#7501=VERTEX_POINT('',#32587);
#7502=VERTEX_POINT('',#32589);
#7503=VERTEX_POINT('',#32591);
#7504=VERTEX_POINT('',#32595);
#7505=VERTEX_POINT('',#32599);
#7506=VERTEX_POINT('',#32603);
#7507=VERTEX_POINT('',#32607);
#7508=VERTEX_POINT('',#32611);
#7509=VERTEX_POINT('',#32615);
#7510=VERTEX_POINT('',#32619);
#7511=VERTEX_POINT('',#32623);
#7512=VERTEX_POINT('',#32627);
#7513=VERTEX_POINT('',#32631);
#7514=VERTEX_POINT('',#32635);
#7515=VERTEX_POINT('',#32637);
#7516=VERTEX_POINT('',#32641);
#7517=VERTEX_POINT('',#32645);
#7518=VERTEX_POINT('',#32649);
#7519=VERTEX_POINT('',#32653);
#7520=VERTEX_POINT('',#32657);
#7521=VERTEX_POINT('',#32661);
#7522=VERTEX_POINT('',#32665);
#7523=VERTEX_POINT('',#32669);
#7524=VERTEX_POINT('',#32673);
#7525=VERTEX_POINT('',#32681);
#7526=VERTEX_POINT('',#32683);
#7527=VERTEX_POINT('',#32685);
#7528=VERTEX_POINT('',#32694);
#7529=VERTEX_POINT('',#32709);
#7530=VERTEX_POINT('',#32711);
#7531=VERTEX_POINT('',#32722);
#7532=VERTEX_POINT('',#32728);
#7533=VERTEX_POINT('',#32732);
#7534=VERTEX_POINT('',#32736);
#7535=VERTEX_POINT('',#32740);
#7536=VERTEX_POINT('',#32744);
#7537=VERTEX_POINT('',#32753);
#7538=VERTEX_POINT('',#32764);
#7539=VERTEX_POINT('',#32770);
#7540=VERTEX_POINT('',#32774);
#7541=VERTEX_POINT('',#32778);
#7542=VERTEX_POINT('',#32787);
#7543=VERTEX_POINT('',#32798);
#7544=VERTEX_POINT('',#32804);
#7545=VERTEX_POINT('',#32808);
#7546=VERTEX_POINT('',#32812);
#7547=VERTEX_POINT('',#32816);
#7548=VERTEX_POINT('',#32823);
#7549=VERTEX_POINT('',#32825);
#7550=VERTEX_POINT('',#32829);
#7551=VERTEX_POINT('',#32833);
#7552=VERTEX_POINT('',#32837);
#7553=VERTEX_POINT('',#32841);
#7554=VERTEX_POINT('',#32845);
#7555=VERTEX_POINT('',#32849);
#7556=VERTEX_POINT('',#32861);
#7557=VERTEX_POINT('',#32863);
#7558=VERTEX_POINT('',#32874);
#7559=VERTEX_POINT('',#32885);
#7560=VERTEX_POINT('',#32896);
#7561=VERTEX_POINT('',#32907);
#7562=VERTEX_POINT('',#32918);
#7563=VERTEX_POINT('',#32929);
#7564=VERTEX_POINT('',#32940);
#7565=VERTEX_POINT('',#32951);
#7566=VERTEX_POINT('',#32962);
#7567=VERTEX_POINT('',#32973);
#7568=VERTEX_POINT('',#32994);
#7569=VERTEX_POINT('',#32996);
#7570=VERTEX_POINT('',#33007);
#7571=VERTEX_POINT('',#33013);
#7572=VERTEX_POINT('',#33022);
#7573=VERTEX_POINT('',#33033);
#7574=VERTEX_POINT('',#33039);
#7575=VERTEX_POINT('',#33043);
#7576=VERTEX_POINT('',#33047);
#7577=VERTEX_POINT('',#33059);
#7578=VERTEX_POINT('',#33061);
#7579=VERTEX_POINT('',#33072);
#7580=VERTEX_POINT('',#33083);
#7581=VERTEX_POINT('',#33094);
#7582=VERTEX_POINT('',#33105);
#7583=VERTEX_POINT('',#33116);
#7584=VERTEX_POINT('',#33127);
#7585=VERTEX_POINT('',#33138);
#7586=VERTEX_POINT('',#33149);
#7587=VERTEX_POINT('',#33160);
#7588=VERTEX_POINT('',#33171);
#7589=VERTEX_POINT('',#33182);
#7590=VERTEX_POINT('',#33188);
#7591=VERTEX_POINT('',#33197);
#7592=VERTEX_POINT('',#33208);
#7593=VERTEX_POINT('',#33219);
#7594=VERTEX_POINT('',#33230);
#7595=VERTEX_POINT('',#33241);
#7596=VERTEX_POINT('',#33252);
#7597=VERTEX_POINT('',#33263);
#7598=VERTEX_POINT('',#33274);
#7599=VERTEX_POINT('',#33285);
#7600=VERTEX_POINT('',#33296);
#7601=VERTEX_POINT('',#33307);
#7602=VERTEX_POINT('',#33313);
#7603=VERTEX_POINT('',#33317);
#7604=VERTEX_POINT('',#33321);
#7605=VERTEX_POINT('',#33325);
#9145=EDGE_CURVE('',#7388,#7389,#4171,.T.);
#9146=EDGE_CURVE('',#7389,#7390,#4172,.T.);
#9147=EDGE_CURVE('',#7390,#7391,#4173,.T.);
#9148=EDGE_CURVE('',#7391,#7388,#4174,.T.);
#9149=EDGE_CURVE('',#7388,#7392,#4175,.T.);
#9150=EDGE_CURVE('',#7393,#7392,#4176,.T.);
#9151=EDGE_CURVE('',#7393,#7394,#4177,.T.);
#9152=EDGE_CURVE('',#7394,#7395,#4178,.T.);
#9153=EDGE_CURVE('',#7395,#7389,#4179,.T.);
#9154=EDGE_CURVE('',#7396,#7391,#4180,.T.);
#9155=EDGE_CURVE('',#7392,#7396,#4181,.T.);
#9156=EDGE_CURVE('',#7397,#7398,#4182,.T.);
#9157=EDGE_CURVE('',#7398,#7399,#4183,.T.);
#9158=EDGE_CURVE('',#7399,#7400,#4184,.T.);
#9159=EDGE_CURVE('',#7400,#7397,#4185,.T.);
#9160=EDGE_CURVE('',#7401,#7400,#4186,.T.);
#9161=EDGE_CURVE('',#7402,#7401,#4187,.T.);
#9162=EDGE_CURVE('',#7397,#7402,#4188,.T.);
#9163=EDGE_CURVE('',#7399,#7395,#4189,.T.);
#9164=EDGE_CURVE('',#7395,#7403,#4190,.T.);
#9165=EDGE_CURVE('',#7403,#7404,#4191,.T.);
#9166=EDGE_CURVE('',#7401,#7404,#4192,.T.);
#9167=EDGE_CURVE('',#7405,#7406,#4193,.T.);
#9168=EDGE_CURVE('',#7406,#7407,#4194,.T.);
#9169=EDGE_CURVE('',#7407,#7408,#4195,.T.);
#9170=EDGE_CURVE('',#7408,#7409,#4196,.T.);
#9171=EDGE_CURVE('',#7409,#7410,#4197,.T.);
#9172=EDGE_CURVE('',#7410,#7405,#4198,.T.);
#9173=EDGE_CURVE('',#7411,#7406,#4199,.T.);
#9174=EDGE_CURVE('',#7412,#7411,#4200,.T.);
#9175=EDGE_CURVE('',#7407,#7412,#4201,.T.);
#9176=EDGE_CURVE('',#7413,#7405,#4202,.T.);
#9177=EDGE_CURVE('',#7413,#7414,#4203,.T.);
#9178=EDGE_CURVE('',#7414,#7415,#4204,.T.);
#9179=EDGE_CURVE('',#7411,#7415,#4205,.T.);
#9180=EDGE_CURVE('',#7410,#7416,#4206,.T.);
#9181=EDGE_CURVE('',#7417,#7416,#4207,.T.);
#9182=EDGE_CURVE('',#7417,#7413,#4208,.T.);
#9183=EDGE_CURVE('',#7418,#7419,#4209,.T.);
#9184=EDGE_CURVE('',#7419,#7420,#4210,.T.);
#9185=EDGE_CURVE('',#7420,#7421,#4211,.T.);
#9186=EDGE_CURVE('',#7421,#7422,#4212,.T.);
#9187=EDGE_CURVE('',#7422,#7418,#4213,.T.);
#9188=EDGE_CURVE('',#7423,#7418,#4214,.T.);
#9189=EDGE_CURVE('',#7422,#7424,#4215,.T.);
#9190=EDGE_CURVE('',#7424,#7423,#4216,.T.);
#9191=EDGE_CURVE('',#7408,#7425,#4217,.T.);
#9192=EDGE_CURVE('',#7425,#7423,#4218,.T.);
#9193=EDGE_CURVE('',#7424,#7409,#4219,.T.);
#9194=EDGE_CURVE('',#7419,#7426,#4220,.T.);
#9195=EDGE_CURVE('',#7426,#7427,#4221,.T.);
#9196=EDGE_CURVE('',#7428,#7427,#4222,.T.);
#9197=EDGE_CURVE('',#7428,#7429,#4223,.T.);
#9198=EDGE_CURVE('',#7420,#7429,#4224,.T.);
#9199=EDGE_CURVE('',#7430,#7425,#4225,.T.);
#9200=EDGE_CURVE('',#7431,#7430,#4226,.T.);
#9201=EDGE_CURVE('',#7432,#7431,#4227,.T.);
#9202=EDGE_CURVE('',#7426,#7432,#4228,.T.);
#9203=EDGE_CURVE('',#7433,#7412,#4229,.T.);
#9204=EDGE_CURVE('',#7433,#7430,#4230,.T.);
#9205=EDGE_CURVE('',#7434,#7435,#4231,.T.);
#9206=EDGE_CURVE('',#7435,#7436,#4232,.T.);
#9207=EDGE_CURVE('',#7436,#7437,#4233,.T.);
#9208=EDGE_CURVE('',#7437,#7434,#4234,.T.);
#9209=EDGE_CURVE('',#7434,#7438,#4235,.T.);
#9210=EDGE_CURVE('',#7439,#7438,#4236,.T.);
#9211=EDGE_CURVE('',#7439,#7414,#4237,.T.);
#9212=EDGE_CURVE('',#7414,#7394,#4238,.T.);
#9213=EDGE_CURVE('',#7394,#7435,#4239,.T.);
#9214=EDGE_CURVE('',#7440,#7437,#4240,.T.);
#9215=EDGE_CURVE('',#7438,#7440,#4241,.T.);
#9216=EDGE_CURVE('',#7396,#7441,#4242,.T.);
#9217=EDGE_CURVE('',#7441,#7393,#4243,.T.);
#9218=EDGE_CURVE('',#7415,#7433,#4244,.T.);
#9219=EDGE_CURVE('',#7442,#7439,#4245,.T.);
#9220=EDGE_CURVE('',#7430,#7442,#4246,.T.);
#9221=EDGE_CURVE('',#7440,#7442,#4247,.T.);
#9222=EDGE_CURVE('',#7443,#7444,#4248,.T.);
#9223=EDGE_CURVE('',#7444,#7445,#4249,.T.);
#9224=EDGE_CURVE('',#7445,#7446,#4250,.T.);
#9225=EDGE_CURVE('',#7446,#7447,#4251,.T.);
#9226=EDGE_CURVE('',#7447,#7443,#4252,.T.);
#9227=EDGE_CURVE('',#7447,#7417,#4253,.T.);
#9228=EDGE_CURVE('',#7416,#7443,#4254,.T.);
#9229=EDGE_CURVE('',#7403,#7446,#4255,.T.);
#9230=EDGE_CURVE('',#7448,#7449,#485,.T.);
#9231=EDGE_CURVE('',#7449,#7450,#4256,.T.);
#9232=EDGE_CURVE('',#7450,#7451,#4257,.T.);
#9233=EDGE_CURVE('',#7451,#7452,#4258,.T.);
#9234=EDGE_CURVE('',#7452,#7453,#4259,.T.);
#9235=EDGE_CURVE('',#7453,#7454,#4260,.T.);
#9236=EDGE_CURVE('',#7454,#7455,#486,.T.);
#9237=EDGE_CURVE('',#7455,#7456,#487,.T.);
#9238=EDGE_CURVE('',#7456,#7457,#4261,.T.);
#9239=EDGE_CURVE('',#7457,#7458,#4262,.T.);
#9240=EDGE_CURVE('',#7458,#7459,#4263,.T.);
#9241=EDGE_CURVE('',#7459,#7460,#488,.T.);
#9242=EDGE_CURVE('',#7460,#7461,#489,.T.);
#9243=EDGE_CURVE('',#7461,#7462,#4264,.T.);
#9244=EDGE_CURVE('',#7462,#7463,#4265,.T.);
#9245=EDGE_CURVE('',#7463,#7464,#4266,.T.);
#9246=EDGE_CURVE('',#7464,#7465,#4267,.T.);
#9247=EDGE_CURVE('',#7465,#7466,#4268,.T.);
#9248=EDGE_CURVE('',#7466,#7448,#490,.T.);
#9249=EDGE_CURVE('',#7467,#7468,#4269,.T.);
#9250=EDGE_CURVE('',#7468,#7469,#4270,.T.);
#9251=EDGE_CURVE('',#7469,#7470,#4271,.T.);
#9252=EDGE_CURVE('',#7470,#7471,#4272,.T.);
#9253=EDGE_CURVE('',#7471,#7472,#4273,.T.);
#9254=EDGE_CURVE('',#7472,#7473,#4274,.T.);
#9255=EDGE_CURVE('',#7473,#7474,#4275,.T.);
#9256=EDGE_CURVE('',#7474,#7467,#4276,.T.);
#9257=EDGE_CURVE('',#7475,#7476,#491,.T.);
#9258=EDGE_CURVE('',#7476,#7477,#492,.T.);
#9259=EDGE_CURVE('',#7477,#7478,#493,.T.);
#9260=EDGE_CURVE('',#7478,#7479,#494,.T.);
#9261=EDGE_CURVE('',#7479,#7480,#495,.T.);
#9262=EDGE_CURVE('',#7480,#7481,#496,.T.);
#9263=EDGE_CURVE('',#7481,#7482,#497,.T.);
#9264=EDGE_CURVE('',#7482,#7483,#498,.T.);
#9265=EDGE_CURVE('',#7483,#7484,#499,.T.);
#9266=EDGE_CURVE('',#7484,#7485,#500,.T.);
#9267=EDGE_CURVE('',#7485,#7486,#501,.T.);
#9268=EDGE_CURVE('',#7486,#7475,#502,.T.);
#9269=EDGE_CURVE('',#7487,#7488,#503,.T.);
#9270=EDGE_CURVE('',#7488,#7489,#4277,.T.);
#9271=EDGE_CURVE('',#7489,#7490,#4278,.T.);
#9272=EDGE_CURVE('',#7490,#7491,#4279,.T.);
#9273=EDGE_CURVE('',#7491,#7492,#4280,.T.);
#9274=EDGE_CURVE('',#7492,#7493,#504,.T.);
#9275=EDGE_CURVE('',#7493,#7494,#505,.T.);
#9276=EDGE_CURVE('',#7494,#7495,#4281,.T.);
#9277=EDGE_CURVE('',#7495,#7487,#506,.T.);
#9278=EDGE_CURVE('',#7496,#7497,#507,.T.);
#9279=EDGE_CURVE('',#7497,#7498,#4282,.T.);
#9280=EDGE_CURVE('',#7498,#7499,#4283,.T.);
#9281=EDGE_CURVE('',#7499,#7500,#4284,.T.);
#9282=EDGE_CURVE('',#7500,#7501,#4285,.T.);
#9283=EDGE_CURVE('',#7501,#7502,#4286,.T.);
#9284=EDGE_CURVE('',#7502,#7503,#508,.T.);
#9285=EDGE_CURVE('',#7503,#7504,#509,.T.);
#9286=EDGE_CURVE('',#7504,#7505,#510,.T.);
#9287=EDGE_CURVE('',#7505,#7506,#511,.T.);
#9288=EDGE_CURVE('',#7506,#7507,#512,.T.);
#9289=EDGE_CURVE('',#7507,#7508,#513,.T.);
#9290=EDGE_CURVE('',#7508,#7509,#514,.T.);
#9291=EDGE_CURVE('',#7509,#7510,#515,.T.);
#9292=EDGE_CURVE('',#7510,#7511,#516,.T.);
#9293=EDGE_CURVE('',#7511,#7512,#517,.T.);
#9294=EDGE_CURVE('',#7512,#7513,#518,.T.);
#9295=EDGE_CURVE('',#7513,#7514,#4287,.T.);
#9296=EDGE_CURVE('',#7514,#7515,#519,.T.);
#9297=EDGE_CURVE('',#7515,#7516,#520,.T.);
#9298=EDGE_CURVE('',#7516,#7517,#521,.T.);
#9299=EDGE_CURVE('',#7517,#7518,#522,.T.);
#9300=EDGE_CURVE('',#7518,#7519,#523,.T.);
#9301=EDGE_CURVE('',#7519,#7520,#524,.T.);
#9302=EDGE_CURVE('',#7520,#7521,#525,.T.);
#9303=EDGE_CURVE('',#7521,#7522,#526,.T.);
#9304=EDGE_CURVE('',#7522,#7523,#527,.T.);
#9305=EDGE_CURVE('',#7523,#7524,#528,.T.);
#9306=EDGE_CURVE('',#7524,#7496,#529,.T.);
#9307=EDGE_CURVE('',#7525,#7445,#4288,.T.);
#9308=EDGE_CURVE('',#7525,#7526,#4289,.T.);
#9309=EDGE_CURVE('',#7527,#7526,#4290,.T.);
#9310=EDGE_CURVE('',#7527,#7403,#4291,.T.);
#9311=EDGE_CURVE('',#7429,#7525,#4292,.T.);
#9312=EDGE_CURVE('',#7444,#7421,#4293,.T.);
#9313=EDGE_CURVE('',#7526,#7428,#4294,.T.);
#9314=EDGE_CURVE('',#7404,#7528,#4295,.T.);
#9315=EDGE_CURVE('',#7528,#7402,#4296,.T.);
#9316=EDGE_CURVE('',#7528,#7426,#4297,.T.);
#9317=EDGE_CURVE('',#7432,#7398,#4298,.T.);
#9318=EDGE_CURVE('',#7427,#7527,#4299,.T.);
#9319=EDGE_CURVE('',#7448,#7529,#4300,.T.);
#9320=EDGE_CURVE('',#7529,#7530,#530,.T.);
#9321=EDGE_CURVE('',#7449,#7530,#4301,.T.);
#9322=EDGE_CURVE('',#7466,#7531,#4302,.T.);
#9323=EDGE_CURVE('',#7531,#7529,#531,.T.);
#9324=EDGE_CURVE('',#7465,#7532,#4303,.T.);
#9325=EDGE_CURVE('',#7532,#7531,#4304,.T.);
#9326=EDGE_CURVE('',#7464,#7533,#4305,.T.);
#9327=EDGE_CURVE('',#7533,#7532,#4306,.T.);
#9328=EDGE_CURVE('',#7463,#7534,#4307,.T.);
#9329=EDGE_CURVE('',#7534,#7533,#4308,.T.);
#9330=EDGE_CURVE('',#7462,#7535,#4309,.T.);
#9331=EDGE_CURVE('',#7535,#7534,#4310,.T.);
#9332=EDGE_CURVE('',#7461,#7536,#4311,.T.);
#9333=EDGE_CURVE('',#7536,#7535,#4312,.T.);
#9334=EDGE_CURVE('',#7460,#7537,#4313,.T.);
#9335=EDGE_CURVE('',#7537,#7536,#532,.T.);
#9336=EDGE_CURVE('',#7459,#7538,#4314,.T.);
#9337=EDGE_CURVE('',#7538,#7537,#533,.T.);
#9338=EDGE_CURVE('',#7458,#7539,#4315,.T.);
#9339=EDGE_CURVE('',#7539,#7538,#4316,.T.);
#9340=EDGE_CURVE('',#7457,#7540,#4317,.T.);
#9341=EDGE_CURVE('',#7540,#7539,#4318,.T.);
#9342=EDGE_CURVE('',#7456,#7541,#4319,.T.);
#9343=EDGE_CURVE('',#7541,#7540,#4320,.T.);
#9344=EDGE_CURVE('',#7455,#7542,#4321,.T.);
#9345=EDGE_CURVE('',#7542,#7541,#534,.T.);
#9346=EDGE_CURVE('',#7454,#7543,#4322,.T.);
#9347=EDGE_CURVE('',#7543,#7542,#535,.T.);
#9348=EDGE_CURVE('',#7453,#7544,#4323,.T.);
#9349=EDGE_CURVE('',#7544,#7543,#4324,.T.);
#9350=EDGE_CURVE('',#7452,#7545,#4325,.T.);
#9351=EDGE_CURVE('',#7545,#7544,#4326,.T.);
#9352=EDGE_CURVE('',#7451,#7546,#4327,.T.);
#9353=EDGE_CURVE('',#7546,#7545,#4328,.T.);
#9354=EDGE_CURVE('',#7450,#7547,#4329,.T.);
#9355=EDGE_CURVE('',#7547,#7546,#4330,.T.);
#9356=EDGE_CURVE('',#7530,#7547,#4331,.T.);
#9357=EDGE_CURVE('',#7467,#7548,#4332,.T.);
#9358=EDGE_CURVE('',#7548,#7549,#4333,.T.);
#9359=EDGE_CURVE('',#7468,#7549,#4334,.T.);
#9360=EDGE_CURVE('',#7474,#7550,#4335,.T.);
#9361=EDGE_CURVE('',#7550,#7548,#4336,.T.);
#9362=EDGE_CURVE('',#7473,#7551,#4337,.T.);
#9363=EDGE_CURVE('',#7551,#7550,#4338,.T.);
#9364=EDGE_CURVE('',#7472,#7552,#4339,.T.);
#9365=EDGE_CURVE('',#7552,#7551,#4340,.T.);
#9366=EDGE_CURVE('',#7471,#7553,#4341,.T.);
#9367=EDGE_CURVE('',#7553,#7552,#4342,.T.);
#9368=EDGE_CURVE('',#7470,#7554,#4343,.T.);
#9369=EDGE_CURVE('',#7554,#7553,#4344,.T.);
#9370=EDGE_CURVE('',#7469,#7555,#4345,.T.);
#9371=EDGE_CURVE('',#7555,#7554,#4346,.T.);
#9372=EDGE_CURVE('',#7549,#7555,#4347,.T.);
#9373=EDGE_CURVE('',#7475,#7556,#4348,.T.);
#9374=EDGE_CURVE('',#7556,#7557,#536,.T.);
#9375=EDGE_CURVE('',#7476,#7557,#4349,.T.);
#9376=EDGE_CURVE('',#7486,#7558,#4350,.T.);
#9377=EDGE_CURVE('',#7558,#7556,#537,.T.);
#9378=EDGE_CURVE('',#7485,#7559,#4351,.T.);
#9379=EDGE_CURVE('',#7559,#7558,#538,.T.);
#9380=EDGE_CURVE('',#7484,#7560,#4352,.T.);
#9381=EDGE_CURVE('',#7560,#7559,#539,.T.);
#9382=EDGE_CURVE('',#7483,#7561,#4353,.T.);
#9383=EDGE_CURVE('',#7561,#7560,#540,.T.);
#9384=EDGE_CURVE('',#7482,#7562,#4354,.T.);
#9385=EDGE_CURVE('',#7562,#7561,#541,.T.);
#9386=EDGE_CURVE('',#7481,#7563,#4355,.T.);
#9387=EDGE_CURVE('',#7563,#7562,#542,.T.);
#9388=EDGE_CURVE('',#7480,#7564,#4356,.T.);
#9389=EDGE_CURVE('',#7564,#7563,#543,.T.);
#9390=EDGE_CURVE('',#7479,#7565,#4357,.T.);
#9391=EDGE_CURVE('',#7565,#7564,#544,.T.);
#9392=EDGE_CURVE('',#7478,#7566,#4358,.T.);
#9393=EDGE_CURVE('',#7566,#7565,#545,.T.);
#9394=EDGE_CURVE('',#7477,#7567,#4359,.T.);
#9395=EDGE_CURVE('',#7567,#7566,#546,.T.);
#9396=EDGE_CURVE('',#7557,#7567,#547,.T.);
#9397=EDGE_CURVE('',#7487,#7568,#4360,.T.);
#9398=EDGE_CURVE('',#7568,#7569,#548,.T.);
#9399=EDGE_CURVE('',#7488,#7569,#4361,.T.);
#9400=EDGE_CURVE('',#7495,#7570,#4362,.T.);
#9401=EDGE_CURVE('',#7570,#7568,#549,.T.);
#9402=EDGE_CURVE('',#7494,#7571,#4363,.T.);
#9403=EDGE_CURVE('',#7571,#7570,#4364,.T.);
#9404=EDGE_CURVE('',#7493,#7572,#4365,.T.);
#9405=EDGE_CURVE('',#7572,#7571,#550,.T.);
#9406=EDGE_CURVE('',#7492,#7573,#4366,.T.);
#9407=EDGE_CURVE('',#7573,#7572,#551,.T.);
#9408=EDGE_CURVE('',#7491,#7574,#4367,.T.);
#9409=EDGE_CURVE('',#7574,#7573,#4368,.T.);
#9410=EDGE_CURVE('',#7490,#7575,#4369,.T.);
#9411=EDGE_CURVE('',#7575,#7574,#4370,.T.);
#9412=EDGE_CURVE('',#7489,#7576,#4371,.T.);
#9413=EDGE_CURVE('',#7576,#7575,#4372,.T.);
#9414=EDGE_CURVE('',#7569,#7576,#4373,.T.);
#9415=EDGE_CURVE('',#7496,#7577,#4374,.T.);
#9416=EDGE_CURVE('',#7577,#7578,#552,.T.);
#9417=EDGE_CURVE('',#7497,#7578,#4375,.T.);
#9418=EDGE_CURVE('',#7524,#7579,#4376,.T.);
#9419=EDGE_CURVE('',#7579,#7577,#553,.T.);
#9420=EDGE_CURVE('',#7523,#7580,#4377,.T.);
#9421=EDGE_CURVE('',#7580,#7579,#554,.T.);
#9422=EDGE_CURVE('',#7522,#7581,#4378,.T.);
#9423=EDGE_CURVE('',#7581,#7580,#555,.T.);
#9424=EDGE_CURVE('',#7521,#7582,#4379,.T.);
#9425=EDGE_CURVE('',#7582,#7581,#556,.T.);
#9426=EDGE_CURVE('',#7520,#7583,#4380,.T.);
#9427=EDGE_CURVE('',#7583,#7582,#557,.T.);
#9428=EDGE_CURVE('',#7519,#7584,#4381,.T.);
#9429=EDGE_CURVE('',#7584,#7583,#558,.T.);
#9430=EDGE_CURVE('',#7518,#7585,#4382,.T.);
#9431=EDGE_CURVE('',#7585,#7584,#559,.T.);
#9432=EDGE_CURVE('',#7517,#7586,#4383,.T.);
#9433=EDGE_CURVE('',#7586,#7585,#560,.T.);
#9434=EDGE_CURVE('',#7516,#7587,#4384,.T.);
#9435=EDGE_CURVE('',#7587,#7586,#561,.T.);
#9436=EDGE_CURVE('',#7515,#7588,#4385,.T.);
#9437=EDGE_CURVE('',#7588,#7587,#562,.T.);
#9438=EDGE_CURVE('',#7514,#7589,#4386,.T.);
#9439=EDGE_CURVE('',#7589,#7588,#563,.T.);
#9440=EDGE_CURVE('',#7513,#7590,#4387,.T.);
#9441=EDGE_CURVE('',#7590,#7589,#4388,.T.);
#9442=EDGE_CURVE('',#7512,#7591,#4389,.T.);
#9443=EDGE_CURVE('',#7591,#7590,#564,.T.);
#9444=EDGE_CURVE('',#7511,#7592,#4390,.T.);
#9445=EDGE_CURVE('',#7592,#7591,#565,.T.);
#9446=EDGE_CURVE('',#7510,#7593,#4391,.T.);
#9447=EDGE_CURVE('',#7593,#7592,#566,.T.);
#9448=EDGE_CURVE('',#7509,#7594,#4392,.T.);
#9449=EDGE_CURVE('',#7594,#7593,#567,.T.);
#9450=EDGE_CURVE('',#7508,#7595,#4393,.T.);
#9451=EDGE_CURVE('',#7595,#7594,#568,.T.);
#9452=EDGE_CURVE('',#7507,#7596,#4394,.T.);
#9453=EDGE_CURVE('',#7596,#7595,#569,.T.);
#9454=EDGE_CURVE('',#7506,#7597,#4395,.T.);
#9455=EDGE_CURVE('',#7597,#7596,#570,.T.);
#9456=EDGE_CURVE('',#7505,#7598,#4396,.T.);
#9457=EDGE_CURVE('',#7598,#7597,#571,.T.);
#9458=EDGE_CURVE('',#7504,#7599,#4397,.T.);
#9459=EDGE_CURVE('',#7599,#7598,#572,.T.);
#9460=EDGE_CURVE('',#7503,#7600,#4398,.T.);
#9461=EDGE_CURVE('',#7600,#7599,#573,.T.);
#9462=EDGE_CURVE('',#7502,#7601,#4399,.T.);
#9463=EDGE_CURVE('',#7601,#7600,#574,.T.);
#9464=EDGE_CURVE('',#7501,#7602,#4400,.T.);
#9465=EDGE_CURVE('',#7602,#7601,#4401,.T.);
#9466=EDGE_CURVE('',#7500,#7603,#4402,.T.);
#9467=EDGE_CURVE('',#7603,#7602,#4403,.T.);
#9468=EDGE_CURVE('',#7499,#7604,#4404,.T.);
#9469=EDGE_CURVE('',#7604,#7603,#4405,.T.);
#9470=EDGE_CURVE('',#7498,#7605,#4406,.T.);
#9471=EDGE_CURVE('',#7605,#7604,#4407,.T.);
#9472=EDGE_CURVE('',#7578,#7605,#4408,.T.);
#9473=EDGE_CURVE('',#7431,#7441,#4409,.T.);
#9474=EDGE_CURVE('',#7436,#7431,#4410,.T.);
#9475=EDGE_CURVE('',#7390,#7432,#4411,.T.);
#9476=EDGE_CURVE('',#7416,#7424,#4412,.T.);
#9477=EDGE_CURVE('',#7443,#7422,#4413,.T.);
#12164=ORIENTED_EDGE('',*,*,#9145,.T.);
#12165=ORIENTED_EDGE('',*,*,#9146,.T.);
#12166=ORIENTED_EDGE('',*,*,#9147,.T.);
#12167=ORIENTED_EDGE('',*,*,#9148,.T.);
#12168=ORIENTED_EDGE('',*,*,#9145,.F.);
#12169=ORIENTED_EDGE('',*,*,#9149,.T.);
#12170=ORIENTED_EDGE('',*,*,#9150,.F.);
#12171=ORIENTED_EDGE('',*,*,#9151,.T.);
#12172=ORIENTED_EDGE('',*,*,#9152,.T.);
#12173=ORIENTED_EDGE('',*,*,#9153,.T.);
#12174=ORIENTED_EDGE('',*,*,#9148,.F.);
#12175=ORIENTED_EDGE('',*,*,#9154,.F.);
#12176=ORIENTED_EDGE('',*,*,#9155,.F.);
#12177=ORIENTED_EDGE('',*,*,#9149,.F.);
#12178=ORIENTED_EDGE('',*,*,#9156,.T.);
#12179=ORIENTED_EDGE('',*,*,#9157,.T.);
#12180=ORIENTED_EDGE('',*,*,#9158,.T.);
#12181=ORIENTED_EDGE('',*,*,#9159,.T.);
#12182=ORIENTED_EDGE('',*,*,#9159,.F.);
#12183=ORIENTED_EDGE('',*,*,#9160,.F.);
#12184=ORIENTED_EDGE('',*,*,#9161,.F.);
#12185=ORIENTED_EDGE('',*,*,#9162,.F.);
#12186=ORIENTED_EDGE('',*,*,#9158,.F.);
#12187=ORIENTED_EDGE('',*,*,#9163,.T.);
#12188=ORIENTED_EDGE('',*,*,#9164,.T.);
#12189=ORIENTED_EDGE('',*,*,#9165,.T.);
#12190=ORIENTED_EDGE('',*,*,#9166,.F.);
#12191=ORIENTED_EDGE('',*,*,#9160,.T.);
#12192=ORIENTED_EDGE('',*,*,#9167,.T.);
#12193=ORIENTED_EDGE('',*,*,#9168,.T.);
#12194=ORIENTED_EDGE('',*,*,#9169,.T.);
#12195=ORIENTED_EDGE('',*,*,#9170,.T.);
#12196=ORIENTED_EDGE('',*,*,#9171,.T.);
#12197=ORIENTED_EDGE('',*,*,#9172,.T.);
#12198=ORIENTED_EDGE('',*,*,#9168,.F.);
#12199=ORIENTED_EDGE('',*,*,#9173,.F.);
#12200=ORIENTED_EDGE('',*,*,#9174,.F.);
#12201=ORIENTED_EDGE('',*,*,#9175,.F.);
#12202=ORIENTED_EDGE('',*,*,#9167,.F.);
#12203=ORIENTED_EDGE('',*,*,#9176,.F.);
#12204=ORIENTED_EDGE('',*,*,#9177,.T.);
#12205=ORIENTED_EDGE('',*,*,#9178,.T.);
#12206=ORIENTED_EDGE('',*,*,#9179,.F.);
#12207=ORIENTED_EDGE('',*,*,#9173,.T.);
#12208=ORIENTED_EDGE('',*,*,#9172,.F.);
#12209=ORIENTED_EDGE('',*,*,#9180,.T.);
#12210=ORIENTED_EDGE('',*,*,#9181,.F.);
#12211=ORIENTED_EDGE('',*,*,#9182,.T.);
#12212=ORIENTED_EDGE('',*,*,#9176,.T.);
#12213=ORIENTED_EDGE('',*,*,#9183,.T.);
#12214=ORIENTED_EDGE('',*,*,#9184,.T.);
#12215=ORIENTED_EDGE('',*,*,#9185,.T.);
#12216=ORIENTED_EDGE('',*,*,#9186,.T.);
#12217=ORIENTED_EDGE('',*,*,#9187,.T.);
#12218=ORIENTED_EDGE('',*,*,#9188,.T.);
#12219=ORIENTED_EDGE('',*,*,#9187,.F.);
#12220=ORIENTED_EDGE('',*,*,#9189,.T.);
#12221=ORIENTED_EDGE('',*,*,#9190,.T.);
#12222=ORIENTED_EDGE('',*,*,#9170,.F.);
#12223=ORIENTED_EDGE('',*,*,#9191,.T.);
#12224=ORIENTED_EDGE('',*,*,#9192,.T.);
#12225=ORIENTED_EDGE('',*,*,#9190,.F.);
#12226=ORIENTED_EDGE('',*,*,#9193,.T.);
#12227=ORIENTED_EDGE('',*,*,#9184,.F.);
#12228=ORIENTED_EDGE('',*,*,#9194,.T.);
#12229=ORIENTED_EDGE('',*,*,#9195,.T.);
#12230=ORIENTED_EDGE('',*,*,#9196,.F.);
#12231=ORIENTED_EDGE('',*,*,#9197,.T.);
#12232=ORIENTED_EDGE('',*,*,#9198,.F.);
#12233=ORIENTED_EDGE('',*,*,#9183,.F.);
#12234=ORIENTED_EDGE('',*,*,#9188,.F.);
#12235=ORIENTED_EDGE('',*,*,#9192,.F.);
#12236=ORIENTED_EDGE('',*,*,#9199,.F.);
#12237=ORIENTED_EDGE('',*,*,#9200,.F.);
#12238=ORIENTED_EDGE('',*,*,#9201,.F.);
#12239=ORIENTED_EDGE('',*,*,#9202,.F.);
#12240=ORIENTED_EDGE('',*,*,#9194,.F.);
#12241=ORIENTED_EDGE('',*,*,#9169,.F.);
#12242=ORIENTED_EDGE('',*,*,#9175,.T.);
#12243=ORIENTED_EDGE('',*,*,#9203,.F.);
#12244=ORIENTED_EDGE('',*,*,#9204,.T.);
#12245=ORIENTED_EDGE('',*,*,#9199,.T.);
#12246=ORIENTED_EDGE('',*,*,#9191,.F.);
#12247=ORIENTED_EDGE('',*,*,#9205,.T.);
#12248=ORIENTED_EDGE('',*,*,#9206,.T.);
#12249=ORIENTED_EDGE('',*,*,#9207,.T.);
#12250=ORIENTED_EDGE('',*,*,#9208,.T.);
#12251=ORIENTED_EDGE('',*,*,#9205,.F.);
#12252=ORIENTED_EDGE('',*,*,#9209,.T.);
#12253=ORIENTED_EDGE('',*,*,#9210,.F.);
#12254=ORIENTED_EDGE('',*,*,#9211,.T.);
#12255=ORIENTED_EDGE('',*,*,#9212,.T.);
#12256=ORIENTED_EDGE('',*,*,#9213,.T.);
#12257=ORIENTED_EDGE('',*,*,#9208,.F.);
#12258=ORIENTED_EDGE('',*,*,#9214,.F.);
#12259=ORIENTED_EDGE('',*,*,#9215,.F.);
#12260=ORIENTED_EDGE('',*,*,#9209,.F.);
#12261=ORIENTED_EDGE('',*,*,#9216,.T.);
#12262=ORIENTED_EDGE('',*,*,#9217,.T.);
#12263=ORIENTED_EDGE('',*,*,#9150,.T.);
#12264=ORIENTED_EDGE('',*,*,#9155,.T.);
#12265=ORIENTED_EDGE('',*,*,#9179,.T.);
#12266=ORIENTED_EDGE('',*,*,#9218,.T.);
#12267=ORIENTED_EDGE('',*,*,#9203,.T.);
#12268=ORIENTED_EDGE('',*,*,#9174,.T.);
#12269=ORIENTED_EDGE('',*,*,#9218,.F.);
#12270=ORIENTED_EDGE('',*,*,#9178,.F.);
#12271=ORIENTED_EDGE('',*,*,#9211,.F.);
#12272=ORIENTED_EDGE('',*,*,#9219,.F.);
#12273=ORIENTED_EDGE('',*,*,#9220,.F.);
#12274=ORIENTED_EDGE('',*,*,#9204,.F.);
#12275=ORIENTED_EDGE('',*,*,#9221,.T.);
#12276=ORIENTED_EDGE('',*,*,#9219,.T.);
#12277=ORIENTED_EDGE('',*,*,#9210,.T.);
#12278=ORIENTED_EDGE('',*,*,#9215,.T.);
#12279=ORIENTED_EDGE('',*,*,#9222,.T.);
#12280=ORIENTED_EDGE('',*,*,#9223,.T.);
#12281=ORIENTED_EDGE('',*,*,#9224,.T.);
#12282=ORIENTED_EDGE('',*,*,#9225,.T.);
#12283=ORIENTED_EDGE('',*,*,#9226,.T.);
#12284=ORIENTED_EDGE('',*,*,#9227,.T.);
#12285=ORIENTED_EDGE('',*,*,#9181,.T.);
#12286=ORIENTED_EDGE('',*,*,#9228,.T.);
#12287=ORIENTED_EDGE('',*,*,#9226,.F.);
#12288=ORIENTED_EDGE('',*,*,#9182,.F.);
#12289=ORIENTED_EDGE('',*,*,#9227,.F.);
#12290=ORIENTED_EDGE('',*,*,#9225,.F.);
#12291=ORIENTED_EDGE('',*,*,#9229,.F.);
#12292=ORIENTED_EDGE('',*,*,#9164,.F.);
#12293=ORIENTED_EDGE('',*,*,#9152,.F.);
#12294=ORIENTED_EDGE('',*,*,#9212,.F.);
#12295=ORIENTED_EDGE('',*,*,#9177,.F.);
#12296=ORIENTED_EDGE('',*,*,#9230,.T.);
#12297=ORIENTED_EDGE('',*,*,#9231,.T.);
#12298=ORIENTED_EDGE('',*,*,#9232,.T.);
#12299=ORIENTED_EDGE('',*,*,#9233,.T.);
#12300=ORIENTED_EDGE('',*,*,#9234,.T.);
#12301=ORIENTED_EDGE('',*,*,#9235,.T.);
#12302=ORIENTED_EDGE('',*,*,#9236,.T.);
#12303=ORIENTED_EDGE('',*,*,#9237,.T.);
#12304=ORIENTED_EDGE('',*,*,#9238,.T.);
#12305=ORIENTED_EDGE('',*,*,#9239,.T.);
#12306=ORIENTED_EDGE('',*,*,#9240,.T.);
#12307=ORIENTED_EDGE('',*,*,#9241,.T.);
#12308=ORIENTED_EDGE('',*,*,#9242,.T.);
#12309=ORIENTED_EDGE('',*,*,#9243,.T.);
#12310=ORIENTED_EDGE('',*,*,#9244,.T.);
#12311=ORIENTED_EDGE('',*,*,#9245,.T.);
#12312=ORIENTED_EDGE('',*,*,#9246,.T.);
#12313=ORIENTED_EDGE('',*,*,#9247,.T.);
#12314=ORIENTED_EDGE('',*,*,#9248,.T.);
#12315=ORIENTED_EDGE('',*,*,#9249,.T.);
#12316=ORIENTED_EDGE('',*,*,#9250,.T.);
#12317=ORIENTED_EDGE('',*,*,#9251,.T.);
#12318=ORIENTED_EDGE('',*,*,#9252,.T.);
#12319=ORIENTED_EDGE('',*,*,#9253,.T.);
#12320=ORIENTED_EDGE('',*,*,#9254,.T.);
#12321=ORIENTED_EDGE('',*,*,#9255,.T.);
#12322=ORIENTED_EDGE('',*,*,#9256,.T.);
#12323=ORIENTED_EDGE('',*,*,#9257,.T.);
#12324=ORIENTED_EDGE('',*,*,#9258,.T.);
#12325=ORIENTED_EDGE('',*,*,#9259,.T.);
#12326=ORIENTED_EDGE('',*,*,#9260,.T.);
#12327=ORIENTED_EDGE('',*,*,#9261,.T.);
#12328=ORIENTED_EDGE('',*,*,#9262,.T.);
#12329=ORIENTED_EDGE('',*,*,#9263,.T.);
#12330=ORIENTED_EDGE('',*,*,#9264,.T.);
#12331=ORIENTED_EDGE('',*,*,#9265,.T.);
#12332=ORIENTED_EDGE('',*,*,#9266,.T.);
#12333=ORIENTED_EDGE('',*,*,#9267,.T.);
#12334=ORIENTED_EDGE('',*,*,#9268,.T.);
#12335=ORIENTED_EDGE('',*,*,#9269,.T.);
#12336=ORIENTED_EDGE('',*,*,#9270,.T.);
#12337=ORIENTED_EDGE('',*,*,#9271,.T.);
#12338=ORIENTED_EDGE('',*,*,#9272,.T.);
#12339=ORIENTED_EDGE('',*,*,#9273,.T.);
#12340=ORIENTED_EDGE('',*,*,#9274,.T.);
#12341=ORIENTED_EDGE('',*,*,#9275,.T.);
#12342=ORIENTED_EDGE('',*,*,#9276,.T.);
#12343=ORIENTED_EDGE('',*,*,#9277,.T.);
#12344=ORIENTED_EDGE('',*,*,#9278,.T.);
#12345=ORIENTED_EDGE('',*,*,#9279,.T.);
#12346=ORIENTED_EDGE('',*,*,#9280,.T.);
#12347=ORIENTED_EDGE('',*,*,#9281,.T.);
#12348=ORIENTED_EDGE('',*,*,#9282,.T.);
#12349=ORIENTED_EDGE('',*,*,#9283,.T.);
#12350=ORIENTED_EDGE('',*,*,#9284,.T.);
#12351=ORIENTED_EDGE('',*,*,#9285,.T.);
#12352=ORIENTED_EDGE('',*,*,#9286,.T.);
#12353=ORIENTED_EDGE('',*,*,#9287,.T.);
#12354=ORIENTED_EDGE('',*,*,#9288,.T.);
#12355=ORIENTED_EDGE('',*,*,#9289,.T.);
#12356=ORIENTED_EDGE('',*,*,#9290,.T.);
#12357=ORIENTED_EDGE('',*,*,#9291,.T.);
#12358=ORIENTED_EDGE('',*,*,#9292,.T.);
#12359=ORIENTED_EDGE('',*,*,#9293,.T.);
#12360=ORIENTED_EDGE('',*,*,#9294,.T.);
#12361=ORIENTED_EDGE('',*,*,#9295,.T.);
#12362=ORIENTED_EDGE('',*,*,#9296,.T.);
#12363=ORIENTED_EDGE('',*,*,#9297,.T.);
#12364=ORIENTED_EDGE('',*,*,#9298,.T.);
#12365=ORIENTED_EDGE('',*,*,#9299,.T.);
#12366=ORIENTED_EDGE('',*,*,#9300,.T.);
#12367=ORIENTED_EDGE('',*,*,#9301,.T.);
#12368=ORIENTED_EDGE('',*,*,#9302,.T.);
#12369=ORIENTED_EDGE('',*,*,#9303,.T.);
#12370=ORIENTED_EDGE('',*,*,#9304,.T.);
#12371=ORIENTED_EDGE('',*,*,#9305,.T.);
#12372=ORIENTED_EDGE('',*,*,#9306,.T.);
#12373=ORIENTED_EDGE('',*,*,#9224,.F.);
#12374=ORIENTED_EDGE('',*,*,#9307,.F.);
#12375=ORIENTED_EDGE('',*,*,#9308,.T.);
#12376=ORIENTED_EDGE('',*,*,#9309,.F.);
#12377=ORIENTED_EDGE('',*,*,#9310,.T.);
#12378=ORIENTED_EDGE('',*,*,#9229,.T.);
#12379=ORIENTED_EDGE('',*,*,#9185,.F.);
#12380=ORIENTED_EDGE('',*,*,#9198,.T.);
#12381=ORIENTED_EDGE('',*,*,#9311,.T.);
#12382=ORIENTED_EDGE('',*,*,#9307,.T.);
#12383=ORIENTED_EDGE('',*,*,#9223,.F.);
#12384=ORIENTED_EDGE('',*,*,#9312,.T.);
#12385=ORIENTED_EDGE('',*,*,#9311,.F.);
#12386=ORIENTED_EDGE('',*,*,#9197,.F.);
#12387=ORIENTED_EDGE('',*,*,#9313,.F.);
#12388=ORIENTED_EDGE('',*,*,#9308,.F.);
#12389=ORIENTED_EDGE('',*,*,#9166,.T.);
#12390=ORIENTED_EDGE('',*,*,#9314,.T.);
#12391=ORIENTED_EDGE('',*,*,#9315,.T.);
#12392=ORIENTED_EDGE('',*,*,#9161,.T.);
#12393=ORIENTED_EDGE('',*,*,#9156,.F.);
#12394=ORIENTED_EDGE('',*,*,#9162,.T.);
#12395=ORIENTED_EDGE('',*,*,#9315,.F.);
#12396=ORIENTED_EDGE('',*,*,#9316,.T.);
#12397=ORIENTED_EDGE('',*,*,#9202,.T.);
#12398=ORIENTED_EDGE('',*,*,#9317,.T.);
#12399=ORIENTED_EDGE('',*,*,#9314,.F.);
#12400=ORIENTED_EDGE('',*,*,#9165,.F.);
#12401=ORIENTED_EDGE('',*,*,#9310,.F.);
#12402=ORIENTED_EDGE('',*,*,#9318,.F.);
#12403=ORIENTED_EDGE('',*,*,#9195,.F.);
#12404=ORIENTED_EDGE('',*,*,#9316,.F.);
#12405=ORIENTED_EDGE('',*,*,#9196,.T.);
#12406=ORIENTED_EDGE('',*,*,#9318,.T.);
#12407=ORIENTED_EDGE('',*,*,#9309,.T.);
#12408=ORIENTED_EDGE('',*,*,#9313,.T.);
#12409=ORIENTED_EDGE('',*,*,#9230,.F.);
#12410=ORIENTED_EDGE('',*,*,#9319,.T.);
#12411=ORIENTED_EDGE('',*,*,#9320,.T.);
#12412=ORIENTED_EDGE('',*,*,#9321,.F.);
#12413=ORIENTED_EDGE('',*,*,#9248,.F.);
#12414=ORIENTED_EDGE('',*,*,#9322,.T.);
#12415=ORIENTED_EDGE('',*,*,#9323,.T.);
#12416=ORIENTED_EDGE('',*,*,#9319,.F.);
#12417=ORIENTED_EDGE('',*,*,#9247,.F.);
#12418=ORIENTED_EDGE('',*,*,#9324,.T.);
#12419=ORIENTED_EDGE('',*,*,#9325,.T.);
#12420=ORIENTED_EDGE('',*,*,#9322,.F.);
#12421=ORIENTED_EDGE('',*,*,#9246,.F.);
#12422=ORIENTED_EDGE('',*,*,#9326,.T.);
#12423=ORIENTED_EDGE('',*,*,#9327,.T.);
#12424=ORIENTED_EDGE('',*,*,#9324,.F.);
#12425=ORIENTED_EDGE('',*,*,#9245,.F.);
#12426=ORIENTED_EDGE('',*,*,#9328,.T.);
#12427=ORIENTED_EDGE('',*,*,#9329,.T.);
#12428=ORIENTED_EDGE('',*,*,#9326,.F.);
#12429=ORIENTED_EDGE('',*,*,#9244,.F.);
#12430=ORIENTED_EDGE('',*,*,#9330,.T.);
#12431=ORIENTED_EDGE('',*,*,#9331,.T.);
#12432=ORIENTED_EDGE('',*,*,#9328,.F.);
#12433=ORIENTED_EDGE('',*,*,#9243,.F.);
#12434=ORIENTED_EDGE('',*,*,#9332,.T.);
#12435=ORIENTED_EDGE('',*,*,#9333,.T.);
#12436=ORIENTED_EDGE('',*,*,#9330,.F.);
#12437=ORIENTED_EDGE('',*,*,#9242,.F.);
#12438=ORIENTED_EDGE('',*,*,#9334,.T.);
#12439=ORIENTED_EDGE('',*,*,#9335,.T.);
#12440=ORIENTED_EDGE('',*,*,#9332,.F.);
#12441=ORIENTED_EDGE('',*,*,#9241,.F.);
#12442=ORIENTED_EDGE('',*,*,#9336,.T.);
#12443=ORIENTED_EDGE('',*,*,#9337,.T.);
#12444=ORIENTED_EDGE('',*,*,#9334,.F.);
#12445=ORIENTED_EDGE('',*,*,#9240,.F.);
#12446=ORIENTED_EDGE('',*,*,#9338,.T.);
#12447=ORIENTED_EDGE('',*,*,#9339,.T.);
#12448=ORIENTED_EDGE('',*,*,#9336,.F.);
#12449=ORIENTED_EDGE('',*,*,#9239,.F.);
#12450=ORIENTED_EDGE('',*,*,#9340,.T.);
#12451=ORIENTED_EDGE('',*,*,#9341,.T.);
#12452=ORIENTED_EDGE('',*,*,#9338,.F.);
#12453=ORIENTED_EDGE('',*,*,#9238,.F.);
#12454=ORIENTED_EDGE('',*,*,#9342,.T.);
#12455=ORIENTED_EDGE('',*,*,#9343,.T.);
#12456=ORIENTED_EDGE('',*,*,#9340,.F.);
#12457=ORIENTED_EDGE('',*,*,#9237,.F.);
#12458=ORIENTED_EDGE('',*,*,#9344,.T.);
#12459=ORIENTED_EDGE('',*,*,#9345,.T.);
#12460=ORIENTED_EDGE('',*,*,#9342,.F.);
#12461=ORIENTED_EDGE('',*,*,#9236,.F.);
#12462=ORIENTED_EDGE('',*,*,#9346,.T.);
#12463=ORIENTED_EDGE('',*,*,#9347,.T.);
#12464=ORIENTED_EDGE('',*,*,#9344,.F.);
#12465=ORIENTED_EDGE('',*,*,#9235,.F.);
#12466=ORIENTED_EDGE('',*,*,#9348,.T.);
#12467=ORIENTED_EDGE('',*,*,#9349,.T.);
#12468=ORIENTED_EDGE('',*,*,#9346,.F.);
#12469=ORIENTED_EDGE('',*,*,#9234,.F.);
#12470=ORIENTED_EDGE('',*,*,#9350,.T.);
#12471=ORIENTED_EDGE('',*,*,#9351,.T.);
#12472=ORIENTED_EDGE('',*,*,#9348,.F.);
#12473=ORIENTED_EDGE('',*,*,#9233,.F.);
#12474=ORIENTED_EDGE('',*,*,#9352,.T.);
#12475=ORIENTED_EDGE('',*,*,#9353,.T.);
#12476=ORIENTED_EDGE('',*,*,#9350,.F.);
#12477=ORIENTED_EDGE('',*,*,#9232,.F.);
#12478=ORIENTED_EDGE('',*,*,#9354,.T.);
#12479=ORIENTED_EDGE('',*,*,#9355,.T.);
#12480=ORIENTED_EDGE('',*,*,#9352,.F.);
#12481=ORIENTED_EDGE('',*,*,#9231,.F.);
#12482=ORIENTED_EDGE('',*,*,#9321,.T.);
#12483=ORIENTED_EDGE('',*,*,#9356,.T.);
#12484=ORIENTED_EDGE('',*,*,#9354,.F.);
#12485=ORIENTED_EDGE('',*,*,#9356,.F.);
#12486=ORIENTED_EDGE('',*,*,#9320,.F.);
#12487=ORIENTED_EDGE('',*,*,#9323,.F.);
#12488=ORIENTED_EDGE('',*,*,#9325,.F.);
#12489=ORIENTED_EDGE('',*,*,#9327,.F.);
#12490=ORIENTED_EDGE('',*,*,#9329,.F.);
#12491=ORIENTED_EDGE('',*,*,#9331,.F.);
#12492=ORIENTED_EDGE('',*,*,#9333,.F.);
#12493=ORIENTED_EDGE('',*,*,#9335,.F.);
#12494=ORIENTED_EDGE('',*,*,#9337,.F.);
#12495=ORIENTED_EDGE('',*,*,#9339,.F.);
#12496=ORIENTED_EDGE('',*,*,#9341,.F.);
#12497=ORIENTED_EDGE('',*,*,#9343,.F.);
#12498=ORIENTED_EDGE('',*,*,#9345,.F.);
#12499=ORIENTED_EDGE('',*,*,#9347,.F.);
#12500=ORIENTED_EDGE('',*,*,#9349,.F.);
#12501=ORIENTED_EDGE('',*,*,#9351,.F.);
#12502=ORIENTED_EDGE('',*,*,#9353,.F.);
#12503=ORIENTED_EDGE('',*,*,#9355,.F.);
#12504=ORIENTED_EDGE('',*,*,#9249,.F.);
#12505=ORIENTED_EDGE('',*,*,#9357,.T.);
#12506=ORIENTED_EDGE('',*,*,#9358,.T.);
#12507=ORIENTED_EDGE('',*,*,#9359,.F.);
#12508=ORIENTED_EDGE('',*,*,#9256,.F.);
#12509=ORIENTED_EDGE('',*,*,#9360,.T.);
#12510=ORIENTED_EDGE('',*,*,#9361,.T.);
#12511=ORIENTED_EDGE('',*,*,#9357,.F.);
#12512=ORIENTED_EDGE('',*,*,#9255,.F.);
#12513=ORIENTED_EDGE('',*,*,#9362,.T.);
#12514=ORIENTED_EDGE('',*,*,#9363,.T.);
#12515=ORIENTED_EDGE('',*,*,#9360,.F.);
#12516=ORIENTED_EDGE('',*,*,#9254,.F.);
#12517=ORIENTED_EDGE('',*,*,#9364,.T.);
#12518=ORIENTED_EDGE('',*,*,#9365,.T.);
#12519=ORIENTED_EDGE('',*,*,#9362,.F.);
#12520=ORIENTED_EDGE('',*,*,#9253,.F.);
#12521=ORIENTED_EDGE('',*,*,#9366,.T.);
#12522=ORIENTED_EDGE('',*,*,#9367,.T.);
#12523=ORIENTED_EDGE('',*,*,#9364,.F.);
#12524=ORIENTED_EDGE('',*,*,#9252,.F.);
#12525=ORIENTED_EDGE('',*,*,#9368,.T.);
#12526=ORIENTED_EDGE('',*,*,#9369,.T.);
#12527=ORIENTED_EDGE('',*,*,#9366,.F.);
#12528=ORIENTED_EDGE('',*,*,#9251,.F.);
#12529=ORIENTED_EDGE('',*,*,#9370,.T.);
#12530=ORIENTED_EDGE('',*,*,#9371,.T.);
#12531=ORIENTED_EDGE('',*,*,#9368,.F.);
#12532=ORIENTED_EDGE('',*,*,#9250,.F.);
#12533=ORIENTED_EDGE('',*,*,#9359,.T.);
#12534=ORIENTED_EDGE('',*,*,#9372,.T.);
#12535=ORIENTED_EDGE('',*,*,#9370,.F.);
#12536=ORIENTED_EDGE('',*,*,#9372,.F.);
#12537=ORIENTED_EDGE('',*,*,#9358,.F.);
#12538=ORIENTED_EDGE('',*,*,#9361,.F.);
#12539=ORIENTED_EDGE('',*,*,#9363,.F.);
#12540=ORIENTED_EDGE('',*,*,#9365,.F.);
#12541=ORIENTED_EDGE('',*,*,#9367,.F.);
#12542=ORIENTED_EDGE('',*,*,#9369,.F.);
#12543=ORIENTED_EDGE('',*,*,#9371,.F.);
#12544=ORIENTED_EDGE('',*,*,#9257,.F.);
#12545=ORIENTED_EDGE('',*,*,#9373,.T.);
#12546=ORIENTED_EDGE('',*,*,#9374,.T.);
#12547=ORIENTED_EDGE('',*,*,#9375,.F.);
#12548=ORIENTED_EDGE('',*,*,#9268,.F.);
#12549=ORIENTED_EDGE('',*,*,#9376,.T.);
#12550=ORIENTED_EDGE('',*,*,#9377,.T.);
#12551=ORIENTED_EDGE('',*,*,#9373,.F.);
#12552=ORIENTED_EDGE('',*,*,#9267,.F.);
#12553=ORIENTED_EDGE('',*,*,#9378,.T.);
#12554=ORIENTED_EDGE('',*,*,#9379,.T.);
#12555=ORIENTED_EDGE('',*,*,#9376,.F.);
#12556=ORIENTED_EDGE('',*,*,#9266,.F.);
#12557=ORIENTED_EDGE('',*,*,#9380,.T.);
#12558=ORIENTED_EDGE('',*,*,#9381,.T.);
#12559=ORIENTED_EDGE('',*,*,#9378,.F.);
#12560=ORIENTED_EDGE('',*,*,#9265,.F.);
#12561=ORIENTED_EDGE('',*,*,#9382,.T.);
#12562=ORIENTED_EDGE('',*,*,#9383,.T.);
#12563=ORIENTED_EDGE('',*,*,#9380,.F.);
#12564=ORIENTED_EDGE('',*,*,#9264,.F.);
#12565=ORIENTED_EDGE('',*,*,#9384,.T.);
#12566=ORIENTED_EDGE('',*,*,#9385,.T.);
#12567=ORIENTED_EDGE('',*,*,#9382,.F.);
#12568=ORIENTED_EDGE('',*,*,#9263,.F.);
#12569=ORIENTED_EDGE('',*,*,#9386,.T.);
#12570=ORIENTED_EDGE('',*,*,#9387,.T.);
#12571=ORIENTED_EDGE('',*,*,#9384,.F.);
#12572=ORIENTED_EDGE('',*,*,#9262,.F.);
#12573=ORIENTED_EDGE('',*,*,#9388,.T.);
#12574=ORIENTED_EDGE('',*,*,#9389,.T.);
#12575=ORIENTED_EDGE('',*,*,#9386,.F.);
#12576=ORIENTED_EDGE('',*,*,#9261,.F.);
#12577=ORIENTED_EDGE('',*,*,#9390,.T.);
#12578=ORIENTED_EDGE('',*,*,#9391,.T.);
#12579=ORIENTED_EDGE('',*,*,#9388,.F.);
#12580=ORIENTED_EDGE('',*,*,#9260,.F.);
#12581=ORIENTED_EDGE('',*,*,#9392,.T.);
#12582=ORIENTED_EDGE('',*,*,#9393,.T.);
#12583=ORIENTED_EDGE('',*,*,#9390,.F.);
#12584=ORIENTED_EDGE('',*,*,#9259,.F.);
#12585=ORIENTED_EDGE('',*,*,#9394,.T.);
#12586=ORIENTED_EDGE('',*,*,#9395,.T.);
#12587=ORIENTED_EDGE('',*,*,#9392,.F.);
#12588=ORIENTED_EDGE('',*,*,#9258,.F.);
#12589=ORIENTED_EDGE('',*,*,#9375,.T.);
#12590=ORIENTED_EDGE('',*,*,#9396,.T.);
#12591=ORIENTED_EDGE('',*,*,#9394,.F.);
#12592=ORIENTED_EDGE('',*,*,#9396,.F.);
#12593=ORIENTED_EDGE('',*,*,#9374,.F.);
#12594=ORIENTED_EDGE('',*,*,#9377,.F.);
#12595=ORIENTED_EDGE('',*,*,#9379,.F.);
#12596=ORIENTED_EDGE('',*,*,#9381,.F.);
#12597=ORIENTED_EDGE('',*,*,#9383,.F.);
#12598=ORIENTED_EDGE('',*,*,#9385,.F.);
#12599=ORIENTED_EDGE('',*,*,#9387,.F.);
#12600=ORIENTED_EDGE('',*,*,#9389,.F.);
#12601=ORIENTED_EDGE('',*,*,#9391,.F.);
#12602=ORIENTED_EDGE('',*,*,#9393,.F.);
#12603=ORIENTED_EDGE('',*,*,#9395,.F.);
#12604=ORIENTED_EDGE('',*,*,#9269,.F.);
#12605=ORIENTED_EDGE('',*,*,#9397,.T.);
#12606=ORIENTED_EDGE('',*,*,#9398,.T.);
#12607=ORIENTED_EDGE('',*,*,#9399,.F.);
#12608=ORIENTED_EDGE('',*,*,#9277,.F.);
#12609=ORIENTED_EDGE('',*,*,#9400,.T.);
#12610=ORIENTED_EDGE('',*,*,#9401,.T.);
#12611=ORIENTED_EDGE('',*,*,#9397,.F.);
#12612=ORIENTED_EDGE('',*,*,#9276,.F.);
#12613=ORIENTED_EDGE('',*,*,#9402,.T.);
#12614=ORIENTED_EDGE('',*,*,#9403,.T.);
#12615=ORIENTED_EDGE('',*,*,#9400,.F.);
#12616=ORIENTED_EDGE('',*,*,#9275,.F.);
#12617=ORIENTED_EDGE('',*,*,#9404,.T.);
#12618=ORIENTED_EDGE('',*,*,#9405,.T.);
#12619=ORIENTED_EDGE('',*,*,#9402,.F.);
#12620=ORIENTED_EDGE('',*,*,#9274,.F.);
#12621=ORIENTED_EDGE('',*,*,#9406,.T.);
#12622=ORIENTED_EDGE('',*,*,#9407,.T.);
#12623=ORIENTED_EDGE('',*,*,#9404,.F.);
#12624=ORIENTED_EDGE('',*,*,#9273,.F.);
#12625=ORIENTED_EDGE('',*,*,#9408,.T.);
#12626=ORIENTED_EDGE('',*,*,#9409,.T.);
#12627=ORIENTED_EDGE('',*,*,#9406,.F.);
#12628=ORIENTED_EDGE('',*,*,#9272,.F.);
#12629=ORIENTED_EDGE('',*,*,#9410,.T.);
#12630=ORIENTED_EDGE('',*,*,#9411,.T.);
#12631=ORIENTED_EDGE('',*,*,#9408,.F.);
#12632=ORIENTED_EDGE('',*,*,#9271,.F.);
#12633=ORIENTED_EDGE('',*,*,#9412,.T.);
#12634=ORIENTED_EDGE('',*,*,#9413,.T.);
#12635=ORIENTED_EDGE('',*,*,#9410,.F.);
#12636=ORIENTED_EDGE('',*,*,#9270,.F.);
#12637=ORIENTED_EDGE('',*,*,#9399,.T.);
#12638=ORIENTED_EDGE('',*,*,#9414,.T.);
#12639=ORIENTED_EDGE('',*,*,#9412,.F.);
#12640=ORIENTED_EDGE('',*,*,#9414,.F.);
#12641=ORIENTED_EDGE('',*,*,#9398,.F.);
#12642=ORIENTED_EDGE('',*,*,#9401,.F.);
#12643=ORIENTED_EDGE('',*,*,#9403,.F.);
#12644=ORIENTED_EDGE('',*,*,#9405,.F.);
#12645=ORIENTED_EDGE('',*,*,#9407,.F.);
#12646=ORIENTED_EDGE('',*,*,#9409,.F.);
#12647=ORIENTED_EDGE('',*,*,#9411,.F.);
#12648=ORIENTED_EDGE('',*,*,#9413,.F.);
#12649=ORIENTED_EDGE('',*,*,#9278,.F.);
#12650=ORIENTED_EDGE('',*,*,#9415,.T.);
#12651=ORIENTED_EDGE('',*,*,#9416,.T.);
#12652=ORIENTED_EDGE('',*,*,#9417,.F.);
#12653=ORIENTED_EDGE('',*,*,#9306,.F.);
#12654=ORIENTED_EDGE('',*,*,#9418,.T.);
#12655=ORIENTED_EDGE('',*,*,#9419,.T.);
#12656=ORIENTED_EDGE('',*,*,#9415,.F.);
#12657=ORIENTED_EDGE('',*,*,#9305,.F.);
#12658=ORIENTED_EDGE('',*,*,#9420,.T.);
#12659=ORIENTED_EDGE('',*,*,#9421,.T.);
#12660=ORIENTED_EDGE('',*,*,#9418,.F.);
#12661=ORIENTED_EDGE('',*,*,#9304,.F.);
#12662=ORIENTED_EDGE('',*,*,#9422,.T.);
#12663=ORIENTED_EDGE('',*,*,#9423,.T.);
#12664=ORIENTED_EDGE('',*,*,#9420,.F.);
#12665=ORIENTED_EDGE('',*,*,#9303,.F.);
#12666=ORIENTED_EDGE('',*,*,#9424,.T.);
#12667=ORIENTED_EDGE('',*,*,#9425,.T.);
#12668=ORIENTED_EDGE('',*,*,#9422,.F.);
#12669=ORIENTED_EDGE('',*,*,#9302,.F.);
#12670=ORIENTED_EDGE('',*,*,#9426,.T.);
#12671=ORIENTED_EDGE('',*,*,#9427,.T.);
#12672=ORIENTED_EDGE('',*,*,#9424,.F.);
#12673=ORIENTED_EDGE('',*,*,#9301,.F.);
#12674=ORIENTED_EDGE('',*,*,#9428,.T.);
#12675=ORIENTED_EDGE('',*,*,#9429,.T.);
#12676=ORIENTED_EDGE('',*,*,#9426,.F.);
#12677=ORIENTED_EDGE('',*,*,#9300,.F.);
#12678=ORIENTED_EDGE('',*,*,#9430,.T.);
#12679=ORIENTED_EDGE('',*,*,#9431,.T.);
#12680=ORIENTED_EDGE('',*,*,#9428,.F.);
#12681=ORIENTED_EDGE('',*,*,#9299,.F.);
#12682=ORIENTED_EDGE('',*,*,#9432,.T.);
#12683=ORIENTED_EDGE('',*,*,#9433,.T.);
#12684=ORIENTED_EDGE('',*,*,#9430,.F.);
#12685=ORIENTED_EDGE('',*,*,#9298,.F.);
#12686=ORIENTED_EDGE('',*,*,#9434,.T.);
#12687=ORIENTED_EDGE('',*,*,#9435,.T.);
#12688=ORIENTED_EDGE('',*,*,#9432,.F.);
#12689=ORIENTED_EDGE('',*,*,#9297,.F.);
#12690=ORIENTED_EDGE('',*,*,#9436,.T.);
#12691=ORIENTED_EDGE('',*,*,#9437,.T.);
#12692=ORIENTED_EDGE('',*,*,#9434,.F.);
#12693=ORIENTED_EDGE('',*,*,#9296,.F.);
#12694=ORIENTED_EDGE('',*,*,#9438,.T.);
#12695=ORIENTED_EDGE('',*,*,#9439,.T.);
#12696=ORIENTED_EDGE('',*,*,#9436,.F.);
#12697=ORIENTED_EDGE('',*,*,#9295,.F.);
#12698=ORIENTED_EDGE('',*,*,#9440,.T.);
#12699=ORIENTED_EDGE('',*,*,#9441,.T.);
#12700=ORIENTED_EDGE('',*,*,#9438,.F.);
#12701=ORIENTED_EDGE('',*,*,#9294,.F.);
#12702=ORIENTED_EDGE('',*,*,#9442,.T.);
#12703=ORIENTED_EDGE('',*,*,#9443,.T.);
#12704=ORIENTED_EDGE('',*,*,#9440,.F.);
#12705=ORIENTED_EDGE('',*,*,#9293,.F.);
#12706=ORIENTED_EDGE('',*,*,#9444,.T.);
#12707=ORIENTED_EDGE('',*,*,#9445,.T.);
#12708=ORIENTED_EDGE('',*,*,#9442,.F.);
#12709=ORIENTED_EDGE('',*,*,#9292,.F.);
#12710=ORIENTED_EDGE('',*,*,#9446,.T.);
#12711=ORIENTED_EDGE('',*,*,#9447,.T.);
#12712=ORIENTED_EDGE('',*,*,#9444,.F.);
#12713=ORIENTED_EDGE('',*,*,#9291,.F.);
#12714=ORIENTED_EDGE('',*,*,#9448,.T.);
#12715=ORIENTED_EDGE('',*,*,#9449,.T.);
#12716=ORIENTED_EDGE('',*,*,#9446,.F.);
#12717=ORIENTED_EDGE('',*,*,#9290,.F.);
#12718=ORIENTED_EDGE('',*,*,#9450,.T.);
#12719=ORIENTED_EDGE('',*,*,#9451,.T.);
#12720=ORIENTED_EDGE('',*,*,#9448,.F.);
#12721=ORIENTED_EDGE('',*,*,#9289,.F.);
#12722=ORIENTED_EDGE('',*,*,#9452,.T.);
#12723=ORIENTED_EDGE('',*,*,#9453,.T.);
#12724=ORIENTED_EDGE('',*,*,#9450,.F.);
#12725=ORIENTED_EDGE('',*,*,#9288,.F.);
#12726=ORIENTED_EDGE('',*,*,#9454,.T.);
#12727=ORIENTED_EDGE('',*,*,#9455,.T.);
#12728=ORIENTED_EDGE('',*,*,#9452,.F.);
#12729=ORIENTED_EDGE('',*,*,#9287,.F.);
#12730=ORIENTED_EDGE('',*,*,#9456,.T.);
#12731=ORIENTED_EDGE('',*,*,#9457,.T.);
#12732=ORIENTED_EDGE('',*,*,#9454,.F.);
#12733=ORIENTED_EDGE('',*,*,#9286,.F.);
#12734=ORIENTED_EDGE('',*,*,#9458,.T.);
#12735=ORIENTED_EDGE('',*,*,#9459,.T.);
#12736=ORIENTED_EDGE('',*,*,#9456,.F.);
#12737=ORIENTED_EDGE('',*,*,#9285,.F.);
#12738=ORIENTED_EDGE('',*,*,#9460,.T.);
#12739=ORIENTED_EDGE('',*,*,#9461,.T.);
#12740=ORIENTED_EDGE('',*,*,#9458,.F.);
#12741=ORIENTED_EDGE('',*,*,#9284,.F.);
#12742=ORIENTED_EDGE('',*,*,#9462,.T.);
#12743=ORIENTED_EDGE('',*,*,#9463,.T.);
#12744=ORIENTED_EDGE('',*,*,#9460,.F.);
#12745=ORIENTED_EDGE('',*,*,#9283,.F.);
#12746=ORIENTED_EDGE('',*,*,#9464,.T.);
#12747=ORIENTED_EDGE('',*,*,#9465,.T.);
#12748=ORIENTED_EDGE('',*,*,#9462,.F.);
#12749=ORIENTED_EDGE('',*,*,#9282,.F.);
#12750=ORIENTED_EDGE('',*,*,#9466,.T.);
#12751=ORIENTED_EDGE('',*,*,#9467,.T.);
#12752=ORIENTED_EDGE('',*,*,#9464,.F.);
#12753=ORIENTED_EDGE('',*,*,#9281,.F.);
#12754=ORIENTED_EDGE('',*,*,#9468,.T.);
#12755=ORIENTED_EDGE('',*,*,#9469,.T.);
#12756=ORIENTED_EDGE('',*,*,#9466,.F.);
#12757=ORIENTED_EDGE('',*,*,#9280,.F.);
#12758=ORIENTED_EDGE('',*,*,#9470,.T.);
#12759=ORIENTED_EDGE('',*,*,#9471,.T.);
#12760=ORIENTED_EDGE('',*,*,#9468,.F.);
#12761=ORIENTED_EDGE('',*,*,#9279,.F.);
#12762=ORIENTED_EDGE('',*,*,#9417,.T.);
#12763=ORIENTED_EDGE('',*,*,#9472,.T.);
#12764=ORIENTED_EDGE('',*,*,#9470,.F.);
#12765=ORIENTED_EDGE('',*,*,#9472,.F.);
#12766=ORIENTED_EDGE('',*,*,#9416,.F.);
#12767=ORIENTED_EDGE('',*,*,#9419,.F.);
#12768=ORIENTED_EDGE('',*,*,#9421,.F.);
#12769=ORIENTED_EDGE('',*,*,#9423,.F.);
#12770=ORIENTED_EDGE('',*,*,#9425,.F.);
#12771=ORIENTED_EDGE('',*,*,#9427,.F.);
#12772=ORIENTED_EDGE('',*,*,#9429,.F.);
#12773=ORIENTED_EDGE('',*,*,#9431,.F.);
#12774=ORIENTED_EDGE('',*,*,#9433,.F.);
#12775=ORIENTED_EDGE('',*,*,#9435,.F.);
#12776=ORIENTED_EDGE('',*,*,#9437,.F.);
#12777=ORIENTED_EDGE('',*,*,#9439,.F.);
#12778=ORIENTED_EDGE('',*,*,#9441,.F.);
#12779=ORIENTED_EDGE('',*,*,#9443,.F.);
#12780=ORIENTED_EDGE('',*,*,#9445,.F.);
#12781=ORIENTED_EDGE('',*,*,#9447,.F.);
#12782=ORIENTED_EDGE('',*,*,#9449,.F.);
#12783=ORIENTED_EDGE('',*,*,#9451,.F.);
#12784=ORIENTED_EDGE('',*,*,#9453,.F.);
#12785=ORIENTED_EDGE('',*,*,#9455,.F.);
#12786=ORIENTED_EDGE('',*,*,#9457,.F.);
#12787=ORIENTED_EDGE('',*,*,#9459,.F.);
#12788=ORIENTED_EDGE('',*,*,#9461,.F.);
#12789=ORIENTED_EDGE('',*,*,#9463,.F.);
#12790=ORIENTED_EDGE('',*,*,#9465,.F.);
#12791=ORIENTED_EDGE('',*,*,#9467,.F.);
#12792=ORIENTED_EDGE('',*,*,#9469,.F.);
#12793=ORIENTED_EDGE('',*,*,#9471,.F.);
#12794=ORIENTED_EDGE('',*,*,#9206,.F.);
#12795=ORIENTED_EDGE('',*,*,#9213,.F.);
#12796=ORIENTED_EDGE('',*,*,#9151,.F.);
#12797=ORIENTED_EDGE('',*,*,#9217,.F.);
#12798=ORIENTED_EDGE('',*,*,#9473,.F.);
#12799=ORIENTED_EDGE('',*,*,#9474,.F.);
#12800=ORIENTED_EDGE('',*,*,#9147,.F.);
#12801=ORIENTED_EDGE('',*,*,#9475,.T.);
#12802=ORIENTED_EDGE('',*,*,#9201,.T.);
#12803=ORIENTED_EDGE('',*,*,#9473,.T.);
#12804=ORIENTED_EDGE('',*,*,#9216,.F.);
#12805=ORIENTED_EDGE('',*,*,#9154,.T.);
#12806=ORIENTED_EDGE('',*,*,#9207,.F.);
#12807=ORIENTED_EDGE('',*,*,#9474,.T.);
#12808=ORIENTED_EDGE('',*,*,#9200,.T.);
#12809=ORIENTED_EDGE('',*,*,#9220,.T.);
#12810=ORIENTED_EDGE('',*,*,#9221,.F.);
#12811=ORIENTED_EDGE('',*,*,#9214,.T.);
#12812=ORIENTED_EDGE('',*,*,#9171,.F.);
#12813=ORIENTED_EDGE('',*,*,#9193,.F.);
#12814=ORIENTED_EDGE('',*,*,#9476,.F.);
#12815=ORIENTED_EDGE('',*,*,#9180,.F.);
#12816=ORIENTED_EDGE('',*,*,#9146,.F.);
#12817=ORIENTED_EDGE('',*,*,#9153,.F.);
#12818=ORIENTED_EDGE('',*,*,#9163,.F.);
#12819=ORIENTED_EDGE('',*,*,#9157,.F.);
#12820=ORIENTED_EDGE('',*,*,#9317,.F.);
#12821=ORIENTED_EDGE('',*,*,#9475,.F.);
#12822=ORIENTED_EDGE('',*,*,#9186,.F.);
#12823=ORIENTED_EDGE('',*,*,#9312,.F.);
#12824=ORIENTED_EDGE('',*,*,#9222,.F.);
#12825=ORIENTED_EDGE('',*,*,#9477,.T.);
#12826=ORIENTED_EDGE('',*,*,#9189,.F.);
#12827=ORIENTED_EDGE('',*,*,#9477,.F.);
#12828=ORIENTED_EDGE('',*,*,#9228,.F.);
#12829=ORIENTED_EDGE('',*,*,#9476,.T.);
#15829=ADVANCED_FACE('',(#2101),#1136,.T.);
#15830=ADVANCED_FACE('',(#2102),#1137,.T.);
#15831=ADVANCED_FACE('',(#2103),#1138,.T.);
#15832=ADVANCED_FACE('',(#2104),#1139,.T.);
#15833=ADVANCED_FACE('',(#2105),#1140,.T.);
#15834=ADVANCED_FACE('',(#2106),#1141,.T.);
#15835=ADVANCED_FACE('',(#2107),#1142,.T.);
#15836=ADVANCED_FACE('',(#2108),#1143,.T.);
#15837=ADVANCED_FACE('',(#2109),#1144,.T.);
#15838=ADVANCED_FACE('',(#2110),#1145,.T.);
#15839=ADVANCED_FACE('',(#2111),#1146,.T.);
#15840=ADVANCED_FACE('',(#2112),#1147,.T.);
#15841=ADVANCED_FACE('',(#2113),#1148,.T.);
#15842=ADVANCED_FACE('',(#2114),#1149,.T.);
#15843=ADVANCED_FACE('',(#2115),#1150,.T.);
#15844=ADVANCED_FACE('',(#2116),#1151,.T.);
#15845=ADVANCED_FACE('',(#2117),#1152,.T.);
#15846=ADVANCED_FACE('',(#2118),#1153,.T.);
#15847=ADVANCED_FACE('',(#2119),#1154,.T.);
#15848=ADVANCED_FACE('',(#2120),#1155,.T.);
#15849=ADVANCED_FACE('',(#2121),#1156,.T.);
#15850=ADVANCED_FACE('',(#2122),#1157,.T.);
#15851=ADVANCED_FACE('',(#2123),#1158,.T.);
#15852=ADVANCED_FACE('',(#2124),#1159,.T.);
#15853=ADVANCED_FACE('',(#2125),#1160,.T.);
#15854=ADVANCED_FACE('',(#2126,#965,#966,#967,#968,#969),#1161,.F.);
#15855=ADVANCED_FACE('',(#2127),#1162,.T.);
#15856=ADVANCED_FACE('',(#2128),#1163,.T.);
#15857=ADVANCED_FACE('',(#2129),#1164,.T.);
#15858=ADVANCED_FACE('',(#2130),#1165,.T.);
#15859=ADVANCED_FACE('',(#2131),#1166,.T.);
#15860=ADVANCED_FACE('',(#2132),#1167,.T.);
#15861=ADVANCED_FACE('',(#2133),#1168,.T.);
#15862=ADVANCED_FACE('',(#2134),#858,.F.);
#15863=ADVANCED_FACE('',(#2135),#859,.F.);
#15864=ADVANCED_FACE('',(#2136),#1169,.F.);
#15865=ADVANCED_FACE('',(#2137),#1170,.F.);
#15866=ADVANCED_FACE('',(#2138),#1171,.F.);
#15867=ADVANCED_FACE('',(#2139),#1172,.F.);
#15868=ADVANCED_FACE('',(#2140),#1173,.F.);
#15869=ADVANCED_FACE('',(#2141),#860,.F.);
#15870=ADVANCED_FACE('',(#2142),#861,.F.);
#15871=ADVANCED_FACE('',(#2143),#1174,.F.);
#15872=ADVANCED_FACE('',(#2144),#1175,.F.);
#15873=ADVANCED_FACE('',(#2145),#1176,.F.);
#15874=ADVANCED_FACE('',(#2146),#862,.F.);
#15875=ADVANCED_FACE('',(#2147),#863,.F.);
#15876=ADVANCED_FACE('',(#2148),#1177,.F.);
#15877=ADVANCED_FACE('',(#2149),#1178,.F.);
#15878=ADVANCED_FACE('',(#2150),#1179,.F.);
#15879=ADVANCED_FACE('',(#2151),#1180,.F.);
#15880=ADVANCED_FACE('',(#2152),#1181,.F.);
#15881=ADVANCED_FACE('',(#2153),#1182,.T.);
#15882=ADVANCED_FACE('',(#2154),#1183,.F.);
#15883=ADVANCED_FACE('',(#2155),#1184,.F.);
#15884=ADVANCED_FACE('',(#2156),#1185,.F.);
#15885=ADVANCED_FACE('',(#2157),#1186,.F.);
#15886=ADVANCED_FACE('',(#2158),#1187,.F.);
#15887=ADVANCED_FACE('',(#2159),#1188,.F.);
#15888=ADVANCED_FACE('',(#2160),#1189,.F.);
#15889=ADVANCED_FACE('',(#2161),#1190,.F.);
#15890=ADVANCED_FACE('',(#2162),#1191,.F.);
#15891=ADVANCED_FACE('',(#2163),#864,.F.);
#15892=ADVANCED_FACE('',(#2164),#865,.F.);
#15893=ADVANCED_FACE('',(#2165),#866,.F.);
#15894=ADVANCED_FACE('',(#2166),#867,.F.);
#15895=ADVANCED_FACE('',(#2167),#868,.F.);
#15896=ADVANCED_FACE('',(#2168),#869,.F.);
#15897=ADVANCED_FACE('',(#2169),#870,.F.);
#15898=ADVANCED_FACE('',(#2170),#871,.F.);
#15899=ADVANCED_FACE('',(#2171),#872,.F.);
#15900=ADVANCED_FACE('',(#2172),#873,.F.);
#15901=ADVANCED_FACE('',(#2173),#874,.F.);
#15902=ADVANCED_FACE('',(#2174),#875,.F.);
#15903=ADVANCED_FACE('',(#2175),#1192,.T.);
#15904=ADVANCED_FACE('',(#2176),#876,.F.);
#15905=ADVANCED_FACE('',(#2177),#877,.F.);
#15906=ADVANCED_FACE('',(#2178),#1193,.F.);
#15907=ADVANCED_FACE('',(#2179),#878,.F.);
#15908=ADVANCED_FACE('',(#2180),#879,.F.);
#15909=ADVANCED_FACE('',(#2181),#1194,.F.);
#15910=ADVANCED_FACE('',(#2182),#1195,.F.);
#15911=ADVANCED_FACE('',(#2183),#1196,.F.);
#15912=ADVANCED_FACE('',(#2184),#1197,.F.);
#15913=ADVANCED_FACE('',(#2185),#1198,.T.);
#15914=ADVANCED_FACE('',(#2186),#880,.F.);
#15915=ADVANCED_FACE('',(#2187),#881,.F.);
#15916=ADVANCED_FACE('',(#2188),#882,.F.);
#15917=ADVANCED_FACE('',(#2189),#883,.F.);
#15918=ADVANCED_FACE('',(#2190),#884,.F.);
#15919=ADVANCED_FACE('',(#2191),#885,.F.);
#15920=ADVANCED_FACE('',(#2192),#886,.F.);
#15921=ADVANCED_FACE('',(#2193),#887,.F.);
#15922=ADVANCED_FACE('',(#2194),#888,.F.);
#15923=ADVANCED_FACE('',(#2195),#889,.F.);
#15924=ADVANCED_FACE('',(#2196),#890,.F.);
#15925=ADVANCED_FACE('',(#2197),#891,.F.);
#15926=ADVANCED_FACE('',(#2198),#1199,.F.);
#15927=ADVANCED_FACE('',(#2199),#892,.F.);
#15928=ADVANCED_FACE('',(#2200),#893,.F.);
#15929=ADVANCED_FACE('',(#2201),#894,.F.);
#15930=ADVANCED_FACE('',(#2202),#895,.F.);
#15931=ADVANCED_FACE('',(#2203),#896,.F.);
#15932=ADVANCED_FACE('',(#2204),#897,.F.);
#15933=ADVANCED_FACE('',(#2205),#898,.F.);
#15934=ADVANCED_FACE('',(#2206),#899,.F.);
#15935=ADVANCED_FACE('',(#2207),#900,.F.);
#15936=ADVANCED_FACE('',(#2208),#901,.F.);
#15937=ADVANCED_FACE('',(#2209),#902,.F.);
#15938=ADVANCED_FACE('',(#2210),#1200,.F.);
#15939=ADVANCED_FACE('',(#2211),#1201,.F.);
#15940=ADVANCED_FACE('',(#2212),#1202,.F.);
#15941=ADVANCED_FACE('',(#2213),#1203,.F.);
#15942=ADVANCED_FACE('',(#2214),#1204,.F.);
#15943=ADVANCED_FACE('',(#2215),#1205,.T.);
#15944=ADVANCED_FACE('',(#2216),#1206,.T.);
#15945=ADVANCED_FACE('',(#2217),#1207,.T.);
#15946=ADVANCED_FACE('',(#2218),#1208,.T.);
#15947=ADVANCED_FACE('',(#2219),#1209,.F.);
#15948=ADVANCED_FACE('',(#2220),#1210,.T.);
#15949=ADVANCED_FACE('',(#2221),#1211,.F.);
#15950=ADVANCED_FACE('',(#2222),#1212,.F.);
#16524=CLOSED_SHELL('',(#15829,#15830,#15831,#15832,#15833,#15834,#15835,
#15836,#15837,#15838,#15839,#15840,#15841,#15842,#15843,#15844,#15845,#15846,
#15847,#15848,#15849,#15850,#15851,#15852,#15853,#15854,#15855,#15856,#15857,
#15858,#15859,#15860,#15861,#15862,#15863,#15864,#15865,#15866,#15867,#15868,
#15869,#15870,#15871,#15872,#15873,#15874,#15875,#15876,#15877,#15878,#15879,
#15880,#15881,#15882,#15883,#15884,#15885,#15886,#15887,#15888,#15889,#15890,
#15891,#15892,#15893,#15894,#15895,#15896,#15897,#15898,#15899,#15900,#15901,
#15902,#15903,#15904,#15905,#15906,#15907,#15908,#15909,#15910,#15911,#15912,
#15913,#15914,#15915,#15916,#15917,#15918,#15919,#15920,#15921,#15922,#15923,
#15924,#15925,#15926,#15927,#15928,#15929,#15930,#15931,#15932,#15933,#15934,
#15935,#15936,#15937,#15938,#15939,#15940,#15941,#15942,#15943,#15944,#15945,
#15946,#15947,#15948,#15949,#15950));
#17175=AXIS2_PLACEMENT_3D('',#32264,#19242,#19243);
#17176=AXIS2_PLACEMENT_3D('',#32265,#19244,#19245);
#17177=AXIS2_PLACEMENT_3D('',#32274,#19250,#19251);
#17178=AXIS2_PLACEMENT_3D('',#32284,#19257,#19258);
#17179=AXIS2_PLACEMENT_3D('',#32288,#19261,#19262);
#17180=AXIS2_PLACEMENT_3D('',#32297,#19267,#19268);
#17181=AXIS2_PLACEMENT_3D('',#32303,#19272,#19273);
#17182=AXIS2_PLACEMENT_3D('',#32310,#19278,#19279);
#17183=AXIS2_PLACEMENT_3D('',#32323,#19286,#19287);
#17184=AXIS2_PLACEMENT_3D('',#32329,#19291,#19292);
#17185=AXIS2_PLACEMENT_3D('',#32337,#19297,#19298);
#17186=AXIS2_PLACEMENT_3D('',#32343,#19302,#19303);
#17187=AXIS2_PLACEMENT_3D('',#32354,#19309,#19310);
#17188=AXIS2_PLACEMENT_3D('',#32360,#19314,#19315);
#17189=AXIS2_PLACEMENT_3D('',#32365,#19319,#19320);
#17190=AXIS2_PLACEMENT_3D('',#32375,#19326,#19327);
#17191=AXIS2_PLACEMENT_3D('',#32383,#19332,#19333);
#17192=AXIS2_PLACEMENT_3D('',#32387,#19336,#19337);
#17193=AXIS2_PLACEMENT_3D('',#32396,#19342,#19343);
#17194=AXIS2_PLACEMENT_3D('',#32404,#19349,#19350);
#17195=AXIS2_PLACEMENT_3D('',#32408,#19353,#19354);
#17196=AXIS2_PLACEMENT_3D('',#32412,#19357,#19358);
#17197=AXIS2_PLACEMENT_3D('',#32414,#19360,#19361);
#17198=AXIS2_PLACEMENT_3D('',#32418,#19364,#19365);
#17199=AXIS2_PLACEMENT_3D('',#32420,#19367,#19368);
#17200=AXIS2_PLACEMENT_3D('',#32431,#19374,#19375);
#17201=AXIS2_PLACEMENT_3D('',#32434,#19378,#19379);
#17202=AXIS2_PLACEMENT_3D('',#32680,#19413,#19414);
#17203=AXIS2_PLACEMENT_3D('',#32688,#19419,#19420);
#17204=AXIS2_PLACEMENT_3D('',#32691,#19423,#19424);
#17205=AXIS2_PLACEMENT_3D('',#32693,#19426,#19427);
#17206=AXIS2_PLACEMENT_3D('',#32697,#19430,#19431);
#17207=AXIS2_PLACEMENT_3D('',#32700,#19434,#19435);
#17208=AXIS2_PLACEMENT_3D('',#32702,#19437,#19438);
#17209=AXIS2_PLACEMENT_3D('',#32727,#19442,#19443);
#17210=AXIS2_PLACEMENT_3D('',#32731,#19446,#19447);
#17211=AXIS2_PLACEMENT_3D('',#32735,#19450,#19451);
#17212=AXIS2_PLACEMENT_3D('',#32739,#19454,#19455);
#17213=AXIS2_PLACEMENT_3D('',#32743,#19458,#19459);
#17214=AXIS2_PLACEMENT_3D('',#32769,#19464,#19465);
#17215=AXIS2_PLACEMENT_3D('',#32773,#19468,#19469);
#17216=AXIS2_PLACEMENT_3D('',#32777,#19472,#19473);
#17217=AXIS2_PLACEMENT_3D('',#32803,#19478,#19479);
#17218=AXIS2_PLACEMENT_3D('',#32807,#19482,#19483);
#17219=AXIS2_PLACEMENT_3D('',#32811,#19486,#19487);
#17220=AXIS2_PLACEMENT_3D('',#32815,#19490,#19491);
#17221=AXIS2_PLACEMENT_3D('',#32819,#19494,#19495);
#17222=AXIS2_PLACEMENT_3D('',#32821,#19497,#19498);
#17223=AXIS2_PLACEMENT_3D('',#32822,#19499,#19500);
#17224=AXIS2_PLACEMENT_3D('',#32828,#19504,#19505);
#17225=AXIS2_PLACEMENT_3D('',#32832,#19508,#19509);
#17226=AXIS2_PLACEMENT_3D('',#32836,#19512,#19513);
#17227=AXIS2_PLACEMENT_3D('',#32840,#19516,#19517);
#17228=AXIS2_PLACEMENT_3D('',#32844,#19520,#19521);
#17229=AXIS2_PLACEMENT_3D('',#32848,#19524,#19525);
#17230=AXIS2_PLACEMENT_3D('',#32852,#19528,#19529);
#17231=AXIS2_PLACEMENT_3D('',#32854,#19531,#19532);
#17232=AXIS2_PLACEMENT_3D('',#32987,#19545,#19546);
#17233=AXIS2_PLACEMENT_3D('',#33012,#19550,#19551);
#17234=AXIS2_PLACEMENT_3D('',#33038,#19556,#19557);
#17235=AXIS2_PLACEMENT_3D('',#33042,#19560,#19561);
#17236=AXIS2_PLACEMENT_3D('',#33046,#19564,#19565);
#17237=AXIS2_PLACEMENT_3D('',#33050,#19568,#19569);
#17238=AXIS2_PLACEMENT_3D('',#33052,#19571,#19572);
#17239=AXIS2_PLACEMENT_3D('',#33187,#19586,#19587);
#17240=AXIS2_PLACEMENT_3D('',#33312,#19601,#19602);
#17241=AXIS2_PLACEMENT_3D('',#33316,#19605,#19606);
#17242=AXIS2_PLACEMENT_3D('',#33320,#19609,#19610);
#17243=AXIS2_PLACEMENT_3D('',#33324,#19613,#19614);
#17244=AXIS2_PLACEMENT_3D('',#33328,#19617,#19618);
#17245=AXIS2_PLACEMENT_3D('',#33330,#19620,#19621);
#17246=AXIS2_PLACEMENT_3D('',#33331,#19622,#19623);
#17247=AXIS2_PLACEMENT_3D('',#33334,#19626,#19627);
#17248=AXIS2_PLACEMENT_3D('',#33336,#19629,#19630);
#17249=AXIS2_PLACEMENT_3D('',#33337,#19631,#19632);
#17250=AXIS2_PLACEMENT_3D('',#33339,#19634,#19635);
#17251=AXIS2_PLACEMENT_3D('',#33340,#19636,#19637);
#17252=AXIS2_PLACEMENT_3D('',#33342,#19639,#19640);
#19242=DIRECTION('axis',(0.,0.,1.));
#19243=DIRECTION('refdir',(1.,0.,0.));
#19244=DIRECTION('center_axis',(-0.923879532511287,0.,0.38268343236509));
#19245=DIRECTION('ref_axis',(0.38268343236509,0.,0.923879532511287));
#19246=DIRECTION('',(0.357406744336594,-0.357406744336592,0.862856209461017));
#19247=DIRECTION('',(0.,1.,0.));
#19248=DIRECTION('',(-0.357406744336594,-0.357406744336592,-0.862856209461017));
#19249=DIRECTION('',(0.,-1.,0.));
#19250=DIRECTION('center_axis',(-0.707106781186546,-0.707106781186549,0.));
#19251=DIRECTION('ref_axis',(0.,0.,1.));
#19252=DIRECTION('',(0.,0.,-1.));
#19253=DIRECTION('',(-0.357406744336591,0.357406744336589,0.86285620946102));
#19254=DIRECTION('',(0.577350269189627,-0.577350269189624,-0.577350269189627));
#19255=DIRECTION('',(0.,0.,1.));
#19256=DIRECTION('',(-0.577350269189627,0.577350269189624,-0.577350269189627));
#19257=DIRECTION('center_axis',(-1.,0.,0.));
#19258=DIRECTION('ref_axis',(0.,0.,1.));
#19259=DIRECTION('',(0.,0.,1.));
#19260=DIRECTION('',(0.,1.,0.));
#19261=DIRECTION('center_axis',(-0.382683432365086,0.,0.923879532511288));
#19262=DIRECTION('ref_axis',(0.923879532511288,0.,0.382683432365086));
#19263=DIRECTION('',(-0.86285620946102,0.357406744336589,-0.357406744336591));
#19264=DIRECTION('',(0.,-1.,0.));
#19265=DIRECTION('',(0.86285620946102,0.357406744336589,0.357406744336591));
#19266=DIRECTION('',(0.,1.,0.));
#19267=DIRECTION('center_axis',(0.,0.,1.));
#19268=DIRECTION('ref_axis',(1.,0.,0.));
#19269=DIRECTION('',(-1.,0.,0.));
#19270=DIRECTION('',(0.,-1.,0.));
#19271=DIRECTION('',(1.,0.,0.));
#19272=DIRECTION('center_axis',(0.,-0.707106781186549,0.707106781186546));
#19273=DIRECTION('ref_axis',(1.,0.,0.));
#19274=DIRECTION('',(-0.577350269189627,-0.577350269189624,-0.577350269189627));
#19275=DIRECTION('',(1.,0.,0.));
#19276=DIRECTION('',(-0.577350269189627,0.577350269189624,0.577350269189627));
#19277=DIRECTION('',(0.862856209461016,-0.357406744336594,-0.357406744336595));
#19278=DIRECTION('center_axis',(0.86602540378444,0.,0.499999999999998));
#19279=DIRECTION('ref_axis',(0.499999999999998,0.,-0.86602540378444));
#19280=DIRECTION('',(0.447213595499956,0.447213595499956,-0.774596669241485));
#19281=DIRECTION('',(0.,1.,0.));
#19282=DIRECTION('',(-0.447213595499956,0.447213595499956,0.774596669241485));
#19283=DIRECTION('',(-0.447213595499955,-0.447213595499961,0.774596669241483));
#19284=DIRECTION('',(0.,-1.,0.));
#19285=DIRECTION('',(0.447213595499955,-0.447213595499961,-0.774596669241483));
#19286=DIRECTION('center_axis',(1.,0.,0.));
#19287=DIRECTION('ref_axis',(0.,0.,-1.));
#19288=DIRECTION('',(0.,0.,1.));
#19289=DIRECTION('',(0.,-1.,0.));
#19290=DIRECTION('',(0.,0.,-1.));
#19291=DIRECTION('center_axis',(0.707106781186548,-0.707106781186548,0.));
#19292=DIRECTION('ref_axis',(0.,0.,-1.));
#19293=DIRECTION('',(0.654653670707978,0.654653670707978,0.377964473009226));
#19294=DIRECTION('',(0.,0.,-1.));
#19295=DIRECTION('',(0.577350269189626,0.577350269189626,0.577350269189626));
#19296=DIRECTION('',(-0.357406744336597,-0.357406744336597,-0.862856209461014));
#19297=DIRECTION('center_axis',(0.353553390593274,-0.707106781186547,0.612372435695795));
#19298=DIRECTION('ref_axis',(0.866025403784439,0.,-0.5));
#19299=DIRECTION('',(-0.866025403784439,0.,0.5));
#19300=DIRECTION('',(0.654653670707978,0.654653670707978,0.377964473009226));
#19301=DIRECTION('',(0.866025403784439,0.,-0.5));
#19302=DIRECTION('center_axis',(0.353553390593273,0.707106781186548,-0.612372435695794));
#19303=DIRECTION('ref_axis',(-0.866025403784439,0.,-0.5));
#19304=DIRECTION('',(0.866025403784439,0.,0.5));
#19305=DIRECTION('',(0.654653670707977,-0.654653670707977,-0.377964473009228));
#19306=DIRECTION('',(-0.447213595499961,-0.447213595499955,-0.774596669241483));
#19307=DIRECTION('',(-0.866025403784439,0.,-0.5));
#19308=DIRECTION('',(-0.654653670707977,0.654653670707977,0.377964473009228));
#19309=DIRECTION('center_axis',(0.707106781186548,0.707106781186548,0.));
#19310=DIRECTION('ref_axis',(0.,0.,-1.));
#19311=DIRECTION('',(0.,0.,1.));
#19312=DIRECTION('',(0.,0.,-1.));
#19313=DIRECTION('',(-0.654653670707978,0.654653670707978,-0.377964473009226));
#19314=DIRECTION('center_axis',(0.353553390593274,0.707106781186547,0.612372435695795));
#19315=DIRECTION('ref_axis',(0.866025403784439,0.,-0.5));
#19316=DIRECTION('',(-0.654653670707978,0.654653670707978,-0.377964473009226));
#19317=DIRECTION('',(-0.866025403784439,0.,0.5));
#19318=DIRECTION('',(0.866025403784439,0.,-0.5));
#19319=DIRECTION('center_axis',(0.707106781186548,0.707106781186548,0.));
#19320=DIRECTION('ref_axis',(0.,0.,-1.));
#19321=DIRECTION('',(0.,0.,1.));
#19322=DIRECTION('',(0.577350269189626,-0.577350269189626,-0.577350269189626));
#19323=DIRECTION('',(-0.357406744336593,0.357406744336593,0.862856209461017));
#19324=DIRECTION('',(0.,0.,-1.));
#19325=DIRECTION('',(0.44721359549996,-0.44721359549996,0.774596669241481));
#19326=DIRECTION('center_axis',(0.,1.,0.));
#19327=DIRECTION('ref_axis',(0.,0.,1.));
#19328=DIRECTION('',(0.,0.,1.));
#19329=DIRECTION('',(1.,0.,0.));
#19330=DIRECTION('',(0.,0.,-1.));
#19331=DIRECTION('',(-1.,0.,0.));
#19332=DIRECTION('center_axis',(0.707106781186548,0.707106781186548,0.));
#19333=DIRECTION('ref_axis',(0.,0.,-1.));
#19334=DIRECTION('',(0.357406744336597,-0.357406744336597,0.862856209461014));
#19335=DIRECTION('',(-0.577350269189626,0.577350269189626,-0.577350269189626));
#19336=DIRECTION('center_axis',(-0.382683432365092,0.,-0.923879532511286));
#19337=DIRECTION('ref_axis',(-0.923879532511286,0.,0.382683432365092));
#19338=DIRECTION('',(-0.862856209461016,-0.357406744336594,0.357406744336595));
#19339=DIRECTION('',(0.,1.,0.));
#19340=DIRECTION('',(0.862856209461016,-0.357406744336594,-0.357406744336595));
#19341=DIRECTION('',(0.,-1.,0.));
#19342=DIRECTION('center_axis',(0.,-0.707106781186549,-0.707106781186546));
#19343=DIRECTION('ref_axis',(-1.,0.,0.));
#19344=DIRECTION('',(1.,0.,0.));
#19345=DIRECTION('',(-0.862856209461018,0.357406744336591,-0.357406744336592));
#19346=DIRECTION('',(0.577350269189627,-0.577350269189624,0.577350269189627));
#19347=DIRECTION('',(-1.,0.,0.));
#19348=DIRECTION('',(0.577350269189627,0.577350269189624,-0.577350269189627));
#19349=DIRECTION('center_axis',(0.,0.,-1.));
#19350=DIRECTION('ref_axis',(-1.,0.,0.));
#19351=DIRECTION('',(-1.,0.,0.));
#19352=DIRECTION('',(0.,1.,0.));
#19353=DIRECTION('center_axis',(-0.923879532511288,0.,-0.382683432365086));
#19354=DIRECTION('ref_axis',(-0.382683432365086,0.,0.923879532511288));
#19355=DIRECTION('',(0.357406744336591,0.357406744336589,-0.86285620946102));
#19356=DIRECTION('',(0.,-1.,0.));
#19357=DIRECTION('center_axis',(0.923879532511285,0.,-0.382683432365094));
#19358=DIRECTION('ref_axis',(-0.382683432365094,0.,-0.923879532511285));
#19359=DIRECTION('',(0.,1.,0.));
#19360=DIRECTION('center_axis',(0.707106781186548,0.,-0.707106781186548));
#19361=DIRECTION('ref_axis',(-0.707106781186548,0.,-0.707106781186548));
#19362=DIRECTION('',(0.,-1.,0.));
#19363=DIRECTION('',(-0.577350269189627,-0.577350269189624,-0.577350269189627));
#19364=DIRECTION('center_axis',(0.382683432365088,0.,-0.923879532511287));
#19365=DIRECTION('ref_axis',(-0.923879532511287,0.,-0.382683432365088));
#19366=DIRECTION('',(0.862856209461018,0.357406744336591,0.357406744336592));
#19367=DIRECTION('center_axis',(0.353553390593273,-0.707106781186548,-0.612372435695794));
#19368=DIRECTION('ref_axis',(-0.866025403784439,0.,-0.5));
#19369=DIRECTION('',(0.866025403784439,0.,0.5));
#19370=DIRECTION('',(0.447213595499961,-0.447213595499955,0.774596669241483));
#19371=DIRECTION('',(-0.654653670707977,-0.654653670707977,0.377964473009228));
#19372=DIRECTION('',(-0.866025403784439,0.,-0.5));
#19373=DIRECTION('',(0.654653670707977,0.654653670707977,-0.377964473009228));
#19374=DIRECTION('center_axis',(0.707106781186548,-0.707106781186548,0.));
#19375=DIRECTION('ref_axis',(0.,0.,-1.));
#19376=DIRECTION('',(0.,0.,-1.));
#19377=DIRECTION('',(0.,0.,1.));
#19378=DIRECTION('center_axis',(0.,1.,0.));
#19379=DIRECTION('ref_axis',(1.,0.,0.));
#19380=DIRECTION('',(0.,0.,-1.));
#19381=DIRECTION('',(-0.963357112062784,0.,0.2682220621762));
#19382=DIRECTION('',(0.,0.,1.));
#19383=DIRECTION('',(0.966551553961737,0.,0.256472403065422));
#19384=DIRECTION('',(0.,0.,-1.));
#19385=DIRECTION('',(-0.97411712880263,0.,-0.22604384391821));
#19386=DIRECTION('',(0.962508286041597,0.,-0.271252279808425));
#19387=DIRECTION('',(0.,0.,-1.));
#19388=DIRECTION('',(-0.962206043023297,0.,-0.272322475696461));
#19389=DIRECTION('',(0.97146241747779,0.,-0.237193531590151));
#19390=DIRECTION('',(0.,0.,-1.));
#19391=DIRECTION('',(-0.964398558141811,0.,0.264453060209172));
#19392=DIRECTION('',(0.,0.,1.));
#19393=DIRECTION('',(0.963801688090544,0.,0.266620153090154));
#19394=DIRECTION('',(0.,0.,1.));
#19395=DIRECTION('',(-0.940102113801967,0.,0.340892967990063));
#19396=DIRECTION('',(0.,0.,1.));
#19397=DIRECTION('',(0.933526017108979,0.,-0.358509658699241));
#19398=DIRECTION('',(0.,0.,-1.));
#19399=DIRECTION('',(-0.925486632914917,0.,-0.378780269147971));
#19400=DIRECTION('',(0.,0.,1.));
#19401=DIRECTION('',(0.933183015563907,0.,0.359401529578064));
#19402=DIRECTION('',(0.,0.,-1.));
#19403=DIRECTION('',(-1.,0.,0.));
#19404=DIRECTION('',(0.,0.,1.));
#19405=DIRECTION('',(1.,0.,0.));
#19406=DIRECTION('',(1.,0.,3.11798350272655E-15));
#19407=DIRECTION('',(1.,0.,0.));
#19408=DIRECTION('',(0.,0.,1.));
#19409=DIRECTION('',(1.,0.,0.));
#19410=DIRECTION('',(0.0016102970727879,0.,-0.999998703470828));
#19411=DIRECTION('',(-1.,0.,0.));
#19412=DIRECTION('',(-0.264515837084414,0.,0.964381341550909));
#19413=DIRECTION('center_axis',(0.707106781186548,-0.707106781186548,0.));
#19414=DIRECTION('ref_axis',(0.,0.,-1.));
#19415=DIRECTION('',(-0.44721359549996,-0.44721359549996,-0.774596669241481));
#19416=DIRECTION('',(0.,0.,1.));
#19417=DIRECTION('',(0.357406744336593,0.357406744336593,-0.862856209461017));
#19418=DIRECTION('',(-0.577350269189626,-0.577350269189626,0.577350269189626));
#19419=DIRECTION('center_axis',(0.866025403784437,0.,-0.500000000000003));
#19420=DIRECTION('ref_axis',(-0.500000000000003,0.,-0.866025403784437));
#19421=DIRECTION('',(0.,-1.,0.));
#19422=DIRECTION('',(0.,1.,0.));
#19423=DIRECTION('center_axis',(1.,0.,0.));
#19424=DIRECTION('ref_axis',(0.,0.,-1.));
#19425=DIRECTION('',(0.,1.,0.));
#19426=DIRECTION('center_axis',(0.382683432365092,0.,0.923879532511286));
#19427=DIRECTION('ref_axis',(0.923879532511286,0.,-0.382683432365092));
#19428=DIRECTION('',(0.,1.,0.));
#19429=DIRECTION('',(-0.862856209461016,-0.357406744336594,0.357406744336595));
#19430=DIRECTION('center_axis',(0.,0.707106781186549,0.707106781186546));
#19431=DIRECTION('ref_axis',(1.,0.,0.));
#19432=DIRECTION('',(0.577350269189627,0.577350269189624,-0.577350269189627));
#19433=DIRECTION('',(0.577350269189627,-0.577350269189624,0.577350269189627));
#19434=DIRECTION('center_axis',(0.707106781186548,0.,0.707106781186548));
#19435=DIRECTION('ref_axis',(0.707106781186548,0.,-0.707106781186548));
#19436=DIRECTION('',(0.,-1.,0.));
#19437=DIRECTION('center_axis',(0.923879532511287,0.,0.382683432365089));
#19438=DIRECTION('ref_axis',(0.382683432365089,0.,-0.923879532511287));
#19439=DIRECTION('',(0.,1.,0.));
#19440=DIRECTION('',(0.,1.,0.));
#19441=DIRECTION('',(0.,1.,0.));
#19442=DIRECTION('center_axis',(-0.266620153090154,0.,0.963801688090544));
#19443=DIRECTION('ref_axis',(0.963801688090544,0.,0.266620153090154));
#19444=DIRECTION('',(0.,1.,0.));
#19445=DIRECTION('',(0.963801688090544,0.,0.266620153090154));
#19446=DIRECTION('center_axis',(-1.,0.,0.));
#19447=DIRECTION('ref_axis',(0.,0.,1.));
#19448=DIRECTION('',(0.,1.,0.));
#19449=DIRECTION('',(0.,0.,1.));
#19450=DIRECTION('center_axis',(-0.264453060209172,0.,-0.964398558141811));
#19451=DIRECTION('ref_axis',(-0.964398558141811,0.,0.264453060209172));
#19452=DIRECTION('',(0.,1.,0.));
#19453=DIRECTION('',(-0.964398558141811,0.,0.264453060209172));
#19454=DIRECTION('center_axis',(1.,0.,0.));
#19455=DIRECTION('ref_axis',(0.,0.,-1.));
#19456=DIRECTION('',(0.,1.,0.));
#19457=DIRECTION('',(0.,0.,-1.));
#19458=DIRECTION('center_axis',(0.237193531590151,0.,0.97146241747779));
#19459=DIRECTION('ref_axis',(0.97146241747779,0.,-0.237193531590151));
#19460=DIRECTION('',(0.,1.,0.));
#19461=DIRECTION('',(0.97146241747779,0.,-0.237193531590151));
#19462=DIRECTION('',(0.,1.,0.));
#19463=DIRECTION('',(0.,1.,0.));
#19464=DIRECTION('center_axis',(0.272322475696461,0.,-0.962206043023297));
#19465=DIRECTION('ref_axis',(-0.962206043023297,0.,-0.272322475696461));
#19466=DIRECTION('',(0.,1.,0.));
#19467=DIRECTION('',(-0.962206043023297,0.,-0.272322475696461));
#19468=DIRECTION('center_axis',(1.,0.,0.));
#19469=DIRECTION('ref_axis',(0.,0.,-1.));
#19470=DIRECTION('',(0.,1.,0.));
#19471=DIRECTION('',(0.,0.,-1.));
#19472=DIRECTION('center_axis',(0.271252279808425,0.,0.962508286041597));
#19473=DIRECTION('ref_axis',(0.962508286041597,0.,-0.271252279808425));
#19474=DIRECTION('',(0.,1.,0.));
#19475=DIRECTION('',(0.962508286041597,0.,-0.271252279808425));
#19476=DIRECTION('',(0.,1.,0.));
#19477=DIRECTION('',(0.,1.,0.));
#19478=DIRECTION('center_axis',(0.22604384391821,0.,-0.97411712880263));
#19479=DIRECTION('ref_axis',(-0.97411712880263,0.,-0.22604384391821));
#19480=DIRECTION('',(0.,1.,0.));
#19481=DIRECTION('',(-0.97411712880263,0.,-0.22604384391821));
#19482=DIRECTION('center_axis',(1.,0.,0.));
#19483=DIRECTION('ref_axis',(0.,0.,-1.));
#19484=DIRECTION('',(0.,1.,0.));
#19485=DIRECTION('',(0.,0.,-1.));
#19486=DIRECTION('center_axis',(-0.256472403065422,0.,0.966551553961737));
#19487=DIRECTION('ref_axis',(0.966551553961737,0.,0.256472403065422));
#19488=DIRECTION('',(0.,1.,0.));
#19489=DIRECTION('',(0.966551553961737,0.,0.256472403065422));
#19490=DIRECTION('center_axis',(-1.,0.,0.));
#19491=DIRECTION('ref_axis',(0.,0.,1.));
#19492=DIRECTION('',(0.,1.,0.));
#19493=DIRECTION('',(0.,0.,1.));
#19494=DIRECTION('center_axis',(-0.2682220621762,0.,-0.963357112062784));
#19495=DIRECTION('ref_axis',(-0.963357112062784,0.,0.2682220621762));
#19496=DIRECTION('',(-0.963357112062784,0.,0.2682220621762));
#19497=DIRECTION('center_axis',(0.,-1.,0.));
#19498=DIRECTION('ref_axis',(-1.,0.,0.));
#19499=DIRECTION('center_axis',(-1.,0.,0.));
#19500=DIRECTION('ref_axis',(0.,0.,1.));
#19501=DIRECTION('',(0.,1.,0.));
#19502=DIRECTION('',(0.,0.,1.));
#19503=DIRECTION('',(0.,1.,0.));
#19504=DIRECTION('center_axis',(-0.359401529578064,0.,0.933183015563908));
#19505=DIRECTION('ref_axis',(0.933183015563907,0.,0.359401529578064));
#19506=DIRECTION('',(0.,1.,0.));
#19507=DIRECTION('',(0.933183015563907,0.,0.359401529578064));
#19508=DIRECTION('center_axis',(-1.,0.,0.));
#19509=DIRECTION('ref_axis',(0.,0.,1.));
#19510=DIRECTION('',(0.,1.,0.));
#19511=DIRECTION('',(0.,0.,1.));
#19512=DIRECTION('center_axis',(0.378780269147971,0.,-0.925486632914917));
#19513=DIRECTION('ref_axis',(-0.925486632914917,0.,-0.378780269147971));
#19514=DIRECTION('',(0.,1.,0.));
#19515=DIRECTION('',(-0.925486632914917,0.,-0.378780269147971));
#19516=DIRECTION('center_axis',(1.,0.,0.));
#19517=DIRECTION('ref_axis',(0.,0.,-1.));
#19518=DIRECTION('',(0.,1.,0.));
#19519=DIRECTION('',(0.,0.,-1.));
#19520=DIRECTION('center_axis',(0.358509658699241,0.,0.933526017108979));
#19521=DIRECTION('ref_axis',(0.933526017108979,0.,-0.358509658699241));
#19522=DIRECTION('',(0.,1.,0.));
#19523=DIRECTION('',(0.933526017108979,0.,-0.358509658699241));
#19524=DIRECTION('center_axis',(-1.,0.,0.));
#19525=DIRECTION('ref_axis',(0.,0.,1.));
#19526=DIRECTION('',(0.,1.,0.));
#19527=DIRECTION('',(0.,0.,1.));
#19528=DIRECTION('center_axis',(-0.340892967990063,0.,-0.940102113801967));
#19529=DIRECTION('ref_axis',(-0.940102113801967,0.,0.340892967990063));
#19530=DIRECTION('',(-0.940102113801967,0.,0.340892967990063));
#19531=DIRECTION('center_axis',(0.,1.,0.));
#19532=DIRECTION('ref_axis',(0.,0.,1.));
#19533=DIRECTION('',(0.,1.,0.));
#19534=DIRECTION('',(0.,1.,0.));
#19535=DIRECTION('',(0.,1.,0.));
#19536=DIRECTION('',(0.,1.,0.));
#19537=DIRECTION('',(0.,1.,0.));
#19538=DIRECTION('',(0.,1.,0.));
#19539=DIRECTION('',(0.,1.,0.));
#19540=DIRECTION('',(0.,1.,0.));
#19541=DIRECTION('',(0.,1.,0.));
#19542=DIRECTION('',(0.,1.,0.));
#19543=DIRECTION('',(0.,1.,0.));
#19544=DIRECTION('',(0.,1.,0.));
#19545=DIRECTION('center_axis',(0.,-1.,0.));
#19546=DIRECTION('ref_axis',(-1.,0.,0.));
#19547=DIRECTION('',(0.,1.,0.));
#19548=DIRECTION('',(0.,1.,0.));
#19549=DIRECTION('',(0.,1.,0.));
#19550=DIRECTION('center_axis',(-3.11798350272655E-15,0.,1.));
#19551=DIRECTION('ref_axis',(1.,0.,3.11798350272655E-15));
#19552=DIRECTION('',(0.,1.,0.));
#19553=DIRECTION('',(1.,0.,3.11798350272655E-15));
#19554=DIRECTION('',(0.,1.,0.));
#19555=DIRECTION('',(0.,1.,0.));
#19556=DIRECTION('center_axis',(0.,0.,1.));
#19557=DIRECTION('ref_axis',(1.,0.,0.));
#19558=DIRECTION('',(0.,1.,0.));
#19559=DIRECTION('',(1.,0.,0.));
#19560=DIRECTION('center_axis',(-1.,0.,0.));
#19561=DIRECTION('ref_axis',(0.,0.,1.));
#19562=DIRECTION('',(0.,1.,0.));
#19563=DIRECTION('',(0.,0.,1.));
#19564=DIRECTION('center_axis',(0.,0.,-1.));
#19565=DIRECTION('ref_axis',(-1.,0.,0.));
#19566=DIRECTION('',(0.,1.,0.));
#19567=DIRECTION('',(-1.,0.,0.));
#19568=DIRECTION('center_axis',(1.,0.,0.));
#19569=DIRECTION('ref_axis',(0.,0.,-1.));
#19570=DIRECTION('',(0.,0.,-1.));
#19571=DIRECTION('center_axis',(0.,-1.,0.));
#19572=DIRECTION('ref_axis',(-1.,0.,0.));
#19573=DIRECTION('',(0.,1.,0.));
#19574=DIRECTION('',(0.,1.,0.));
#19575=DIRECTION('',(0.,1.,0.));
#19576=DIRECTION('',(0.,1.,0.));
#19577=DIRECTION('',(0.,1.,0.));
#19578=DIRECTION('',(0.,1.,0.));
#19579=DIRECTION('',(0.,1.,0.));
#19580=DIRECTION('',(0.,1.,0.));
#19581=DIRECTION('',(0.,1.,0.));
#19582=DIRECTION('',(0.,1.,0.));
#19583=DIRECTION('',(0.,1.,0.));
#19584=DIRECTION('',(0.,1.,0.));
#19585=DIRECTION('',(0.,1.,0.));
#19586=DIRECTION('center_axis',(-0.964381341550909,0.,-0.264515837084414));
#19587=DIRECTION('ref_axis',(-0.264515837084414,0.,0.964381341550909));
#19588=DIRECTION('',(0.,1.,0.));
#19589=DIRECTION('',(-0.264515837084414,0.,0.964381341550909));
#19590=DIRECTION('',(0.,1.,0.));
#19591=DIRECTION('',(0.,1.,0.));
#19592=DIRECTION('',(0.,1.,0.));
#19593=DIRECTION('',(0.,1.,0.));
#19594=DIRECTION('',(0.,1.,0.));
#19595=DIRECTION('',(0.,1.,0.));
#19596=DIRECTION('',(0.,1.,0.));
#19597=DIRECTION('',(0.,1.,0.));
#19598=DIRECTION('',(0.,1.,0.));
#19599=DIRECTION('',(0.,1.,0.));
#19600=DIRECTION('',(0.,1.,0.));
#19601=DIRECTION('center_axis',(0.,0.,-1.));
#19602=DIRECTION('ref_axis',(-1.,0.,0.));
#19603=DIRECTION('',(0.,1.,0.));
#19604=DIRECTION('',(-1.,0.,0.));
#19605=DIRECTION('center_axis',(0.999998703470828,0.,0.0016102970727879));
#19606=DIRECTION('ref_axis',(0.0016102970727879,0.,-0.999998703470828));
#19607=DIRECTION('',(0.,1.,0.));
#19608=DIRECTION('',(0.0016102970727879,0.,-0.999998703470828));
#19609=DIRECTION('center_axis',(0.,0.,1.));
#19610=DIRECTION('ref_axis',(1.,0.,0.));
#19611=DIRECTION('',(0.,1.,0.));
#19612=DIRECTION('',(1.,0.,0.));
#19613=DIRECTION('center_axis',(-1.,0.,0.));
#19614=DIRECTION('ref_axis',(0.,0.,1.));
#19615=DIRECTION('',(0.,1.,0.));
#19616=DIRECTION('',(0.,0.,1.));
#19617=DIRECTION('center_axis',(0.,0.,1.));
#19618=DIRECTION('ref_axis',(1.,0.,0.));
#19619=DIRECTION('',(1.,0.,0.));
#19620=DIRECTION('center_axis',(0.,-1.,0.));
#19621=DIRECTION('ref_axis',(-1.,0.,0.));
#19622=DIRECTION('center_axis',(-0.707106781186548,0.,-0.707106781186548));
#19623=DIRECTION('ref_axis',(-0.707106781186548,0.,0.707106781186548));
#19624=DIRECTION('',(-0.577350269189627,-0.577350269189624,0.577350269189627));
#19625=DIRECTION('',(-0.577350269189627,0.577350269189624,0.577350269189627));
#19626=DIRECTION('center_axis',(-0.707106781186546,0.707106781186549,0.));
#19627=DIRECTION('ref_axis',(0.,0.,1.));
#19628=DIRECTION('',(0.577350269189627,0.577350269189624,0.577350269189627));
#19629=DIRECTION('center_axis',(0.,0.707106781186549,-0.707106781186546));
#19630=DIRECTION('ref_axis',(-1.,0.,0.));
#19631=DIRECTION('center_axis',(-0.5,0.,-0.866025403784439));
#19632=DIRECTION('ref_axis',(-0.866025403784439,0.,0.5));
#19633=DIRECTION('',(0.,1.,0.));
#19634=DIRECTION('center_axis',(-0.707106781186548,0.,0.707106781186548));
#19635=DIRECTION('ref_axis',(0.707106781186548,0.,0.707106781186548));
#19636=DIRECTION('center_axis',(-0.5,0.,0.866025403784439));
#19637=DIRECTION('ref_axis',(0.866025403784439,0.,0.5));
#19638=DIRECTION('',(0.,1.,0.));
#19639=DIRECTION('center_axis',(-1.,0.,0.));
#19640=DIRECTION('ref_axis',(0.,0.,1.));
#32264=CARTESIAN_POINT('',(0.,0.,0.));
#32265=CARTESIAN_POINT('Origin',(15.1767766952966,-15.,17.9267766952966));
#32266=CARTESIAN_POINT('',(15.,-14.5,17.5));
#32267=CARTESIAN_POINT('',(15.3535533905933,-14.8535533905933,18.3535533905933));
#32268=CARTESIAN_POINT('',(10.9776939607821,-10.4776939607822,7.78929420810503));
#32269=CARTESIAN_POINT('',(15.3535533905933,14.8535533905933,18.3535533905933));
#32270=CARTESIAN_POINT('',(15.3535533905933,-15.,18.3535533905933));
#32271=CARTESIAN_POINT('',(15.,14.5,17.5));
#32272=CARTESIAN_POINT('',(9.06160024732289,8.56160024732292,3.16343477829391));
#32273=CARTESIAN_POINT('',(15.,-15.,17.5));
#32274=CARTESIAN_POINT('Origin',(15.25,-14.75,-9.5));
#32275=CARTESIAN_POINT('',(15.,-14.5,-17.5));
#32276=CARTESIAN_POINT('',(15.,-14.5,-9.5));
#32277=CARTESIAN_POINT('',(15.3535533905933,-14.8535533905933,-18.3535533905933));
#32278=CARTESIAN_POINT('',(13.9074049329959,-13.4074049329959,-14.8622421710566));
#32279=CARTESIAN_POINT('',(15.5,-15.,-18.5));
#32280=CARTESIAN_POINT('',(13.9166666666667,-13.4166666666667,-16.9166666666667));
#32281=CARTESIAN_POINT('',(15.5,-15.,18.5));
#32282=CARTESIAN_POINT('',(15.5,-15.,-9.5));
#32283=CARTESIAN_POINT('',(10.75,-10.25,13.75));
#32284=CARTESIAN_POINT('Origin',(15.,-15.,-19.));
#32285=CARTESIAN_POINT('',(15.,14.5,-17.5));
#32286=CARTESIAN_POINT('',(15.,14.5,-9.5));
#32287=CARTESIAN_POINT('',(15.,-15.,-17.5));
#32288=CARTESIAN_POINT('Origin',(16.0732233047034,-15.,18.8232233047034));
#32289=CARTESIAN_POINT('',(16.5,14.5,19.));
#32290=CARTESIAN_POINT('',(15.6464466094067,14.8535533905933,18.6464466094067));
#32291=CARTESIAN_POINT('',(21.7161849536895,12.3393854483354,21.1606145516646));
#32292=CARTESIAN_POINT('',(15.6464466094067,-14.8535533905933,18.6464466094067));
#32293=CARTESIAN_POINT('',(15.6464466094067,-15.,18.6464466094067));
#32294=CARTESIAN_POINT('',(16.5,-14.5,19.));
#32295=CARTESIAN_POINT('',(17.0903255238784,-14.2554791617946,19.2445208382054));
#32296=CARTESIAN_POINT('',(16.5,-15.,19.));
#32297=CARTESIAN_POINT('Origin',(15.,-15.,19.));
#32298=CARTESIAN_POINT('',(29.5,-14.5,19.));
#32299=CARTESIAN_POINT('',(19.,-14.5,19.));
#32300=CARTESIAN_POINT('',(29.5,14.5,19.));
#32301=CARTESIAN_POINT('',(29.5,-15.,19.));
#32302=CARTESIAN_POINT('',(19.,14.5,19.));
#32303=CARTESIAN_POINT('Origin',(19.,-14.75,18.75));
#32304=CARTESIAN_POINT('',(16.1666666666667,-14.3333333333333,19.1666666666667));
#32305=CARTESIAN_POINT('',(30.5,-15.,18.5));
#32306=CARTESIAN_POINT('',(19.,-15.,18.5));
#32307=CARTESIAN_POINT('',(30.3535533905933,-14.8535533905933,18.6464466094067));
#32308=CARTESIAN_POINT('',(28.5,-13.,20.5));
#32309=CARTESIAN_POINT('',(25.9315911232999,-13.0219166471783,20.4780833528217));
#32310=CARTESIAN_POINT('Origin',(30.7834936490539,-15.,-3.58910161513776));
#32311=CARTESIAN_POINT('',(30.7834936490539,-14.7165063509461,-3.58910161513775));
#32312=CARTESIAN_POINT('',(31.,-14.5,-3.96410161513776));
#32313=CARTESIAN_POINT('',(28.4813466520527,-17.0186533479473,0.39833395016048));
#32314=CARTESIAN_POINT('',(31.,14.5,-3.96410161513776));
#32315=CARTESIAN_POINT('',(31.,-15.,-3.96410161513776));
#32316=CARTESIAN_POINT('',(30.7834936490539,14.7165063509461,-3.58910161513775));
#32317=CARTESIAN_POINT('',(31.4813466520527,14.0186533479473,-4.79781847254614));
#32318=CARTESIAN_POINT('',(30.5669872981078,14.5,-3.21410161513776));
#32319=CARTESIAN_POINT('',(27.0901923788647,11.0232050807569,2.80788383248868));
#32320=CARTESIAN_POINT('',(30.5669872981078,-14.5,-3.21410161513776));
#32321=CARTESIAN_POINT('',(30.5669872981078,-15.,-3.21410161513776));
#32322=CARTESIAN_POINT('',(30.0901923788647,-14.0232050807569,-2.38826859021799));
#32323=CARTESIAN_POINT('Origin',(31.,-15.,19.));
#32324=CARTESIAN_POINT('',(31.,-14.5,-17.5));
#32325=CARTESIAN_POINT('',(31.,-14.5,9.5));
#32326=CARTESIAN_POINT('',(31.,14.5,-17.5));
#32327=CARTESIAN_POINT('',(31.,-15.,-17.5));
#32328=CARTESIAN_POINT('',(31.,14.5,9.5));
#32329=CARTESIAN_POINT('Origin',(30.75,-14.75,9.5));
#32330=CARTESIAN_POINT('',(30.5,-15.,-3.75277674973256));
#32331=CARTESIAN_POINT('',(31.8538916194217,-13.6461083805783,-2.97110705880585));
#32332=CARTESIAN_POINT('',(30.5,-15.,-18.5));
#32333=CARTESIAN_POINT('',(30.5,-15.,9.5));
#32334=CARTESIAN_POINT('',(30.6464466094067,-14.8535533905933,-18.3535533905933));
#32335=CARTESIAN_POINT('',(35.25,-10.25,-13.75));
#32336=CARTESIAN_POINT('',(35.0223060392179,-10.4776939607821,-7.7892942081051));
#32337=CARTESIAN_POINT('Origin',(27.125,-14.75,-1.51554445662277));
#32338=CARTESIAN_POINT('',(28.,-14.5,-1.73205080756888));
#32339=CARTESIAN_POINT('',(27.25,-14.5,-1.29903810567666));
#32340=CARTESIAN_POINT('',(27.5,-15.,-2.02072594216369));
#32341=CARTESIAN_POINT('',(27.5,-15.,-2.02072594216369));
#32342=CARTESIAN_POINT('',(27.,-15.,-1.73205080756888));
#32343=CARTESIAN_POINT('Origin',(25.625,14.75,0.649519052838329));
#32344=CARTESIAN_POINT('',(27.5,15.,2.02072594216369));
#32345=CARTESIAN_POINT('',(30.5,15.,3.75277674973257));
#32346=CARTESIAN_POINT('',(25.5,15.,0.866025403784438));
#32347=CARTESIAN_POINT('',(30.7834936490539,14.7165063509461,3.58910161513776));
#32348=CARTESIAN_POINT('',(29.2889655234354,16.2110344765646,4.45196783077506));
#32349=CARTESIAN_POINT('',(30.5669872981078,14.5,3.21410161513775));
#32350=CARTESIAN_POINT('',(26.7901923788646,10.7232050807569,-3.32749907475928));
#32351=CARTESIAN_POINT('',(28.,14.5,1.73205080756888));
#32352=CARTESIAN_POINT('',(25.75,14.5,0.43301270189222));
#32353=CARTESIAN_POINT('',(28.,14.5,1.73205080756888));
#32354=CARTESIAN_POINT('Origin',(27.75,14.75,-0.866025403784439));
#32355=CARTESIAN_POINT('',(27.5,15.,-2.02072594216369));
#32356=CARTESIAN_POINT('',(27.5,15.,-0.866025403784439));
#32357=CARTESIAN_POINT('',(28.,14.5,-1.73205080756888));
#32358=CARTESIAN_POINT('',(28.,14.5,-0.866025403784439));
#32359=CARTESIAN_POINT('',(28.,14.5,-1.73205080756888));
#32360=CARTESIAN_POINT('Origin',(27.125,14.75,-1.51554445662277));
#32361=CARTESIAN_POINT('',(30.5,15.,-3.75277674973256));
#32362=CARTESIAN_POINT('',(31.8538916194217,13.6461083805783,-2.97110705880585));
#32363=CARTESIAN_POINT('',(27.,15.,-1.73205080756888));
#32364=CARTESIAN_POINT('',(27.25,14.5,-1.29903810567666));
#32365=CARTESIAN_POINT('Origin',(30.75,14.75,9.5));
#32366=CARTESIAN_POINT('',(30.5,15.,18.5));
#32367=CARTESIAN_POINT('',(30.5,15.,9.5));
#32368=CARTESIAN_POINT('',(30.6464466094067,14.8535533905933,18.3535533905933));
#32369=CARTESIAN_POINT('',(37.0833333333333,8.41666666666667,11.9166666666667));
#32370=CARTESIAN_POINT('',(31.,14.5,17.5));
#32371=CARTESIAN_POINT('',(34.0086887804634,11.4913112195366,10.2363827412455));
#32372=CARTESIAN_POINT('',(31.,14.5,3.96410161513775));
#32373=CARTESIAN_POINT('',(31.,14.5,9.5));
#32374=CARTESIAN_POINT('',(34.7722431864336,10.7277568135664,10.4978184725462));
#32375=CARTESIAN_POINT('Origin',(23.,15.,0.));
#32376=CARTESIAN_POINT('',(30.5,15.,-18.5));
#32377=CARTESIAN_POINT('',(30.5,15.,9.5));
#32378=CARTESIAN_POINT('',(15.5,15.,-18.5));
#32379=CARTESIAN_POINT('',(27.,15.,-18.5));
#32380=CARTESIAN_POINT('',(15.5,15.,18.5));
#32381=CARTESIAN_POINT('',(15.5,15.,-9.5));
#32382=CARTESIAN_POINT('',(19.,15.,18.5));
#32383=CARTESIAN_POINT('Origin',(30.75,14.75,9.5));
#32384=CARTESIAN_POINT('',(30.6464466094067,14.8535533905933,-18.3535533905933));
#32385=CARTESIAN_POINT('',(36.9383997526772,8.56160024732284,-3.16343477829394));
#32386=CARTESIAN_POINT('',(40.25,5.25000000000001,-8.74999999999999));
#32387=CARTESIAN_POINT('Origin',(16.0732233047034,-15.,-18.8232233047034));
#32388=CARTESIAN_POINT('',(16.5,-14.5,-19.));
#32389=CARTESIAN_POINT('',(15.6464466094067,-14.8535533905933,-18.6464466094067));
#32390=CARTESIAN_POINT('',(20.0684088767001,-13.0219166471783,-20.4780833528217));
#32391=CARTESIAN_POINT('',(15.6464466094067,14.8535533905933,-18.6464466094067));
#32392=CARTESIAN_POINT('',(15.6464466094067,-15.,-18.6464466094067));
#32393=CARTESIAN_POINT('',(16.5,14.5,-19.));
#32394=CARTESIAN_POINT('',(24.6942683065113,11.105822933719,-22.394177066281));
#32395=CARTESIAN_POINT('',(16.5,-15.,-19.));
#32396=CARTESIAN_POINT('Origin',(27.,-14.75,-18.75));
#32397=CARTESIAN_POINT('',(29.5,-14.5,-19.));
#32398=CARTESIAN_POINT('',(27.,-14.5,-19.));
#32399=CARTESIAN_POINT('',(30.3535533905933,-14.8535533905933,-18.6464466094067));
#32400=CARTESIAN_POINT('',(28.9096744761216,-14.2554791617946,-19.2445208382054));
#32401=CARTESIAN_POINT('',(29.8333333333333,-14.3333333333333,-19.1666666666667));
#32402=CARTESIAN_POINT('',(27.,-15.,-18.5));
#32403=CARTESIAN_POINT('',(17.5,-13.,-20.5));
#32404=CARTESIAN_POINT('Origin',(31.,-15.,-19.));
#32405=CARTESIAN_POINT('',(29.5,14.5,-19.));
#32406=CARTESIAN_POINT('',(27.,14.5,-19.));
#32407=CARTESIAN_POINT('',(29.5,-15.,-19.));
#32408=CARTESIAN_POINT('Origin',(15.1767766952966,-15.,-17.9267766952966));
#32409=CARTESIAN_POINT('',(15.3535533905933,14.8535533905933,-18.3535533905933));
#32410=CARTESIAN_POINT('',(11.9913112195367,11.4913112195367,-10.2363827412455));
#32411=CARTESIAN_POINT('',(15.3535533905933,-15.,-18.3535533905933));
#32412=CARTESIAN_POINT('Origin',(30.8232233047034,-15.,-17.9267766952966));
#32413=CARTESIAN_POINT('',(30.6464466094067,-15.,-18.3535533905933));
#32414=CARTESIAN_POINT('Origin',(30.5,-15.,-18.5));
#32415=CARTESIAN_POINT('',(30.3535533905933,14.8535533905933,-18.6464466094067));
#32416=CARTESIAN_POINT('',(30.3535533905933,-15.,-18.6464466094067));
#32417=CARTESIAN_POINT('',(24.8333333333333,9.33333333333336,-24.1666666666667));
#32418=CARTESIAN_POINT('Origin',(29.9267766952966,-15.,-18.8232233047034));
#32419=CARTESIAN_POINT('',(24.2838150463105,12.3393854483353,-21.1606145516647));
#32420=CARTESIAN_POINT('Origin',(25.625,-14.75,0.649519052838329));
#32421=CARTESIAN_POINT('',(28.,-14.5,1.73205080756888));
#32422=CARTESIAN_POINT('',(30.5669872981078,-14.5,3.21410161513775));
#32423=CARTESIAN_POINT('',(25.75,-14.5,0.43301270189222));
#32424=CARTESIAN_POINT('',(30.7834936490539,-14.7165063509461,3.58910161513775));
#32425=CARTESIAN_POINT('',(29.7901923788647,-13.7232050807569,1.86865334794731));
#32426=CARTESIAN_POINT('',(30.5,-15.,3.75277674973257));
#32427=CARTESIAN_POINT('',(29.2889655234354,-16.2110344765646,4.45196783077506));
#32428=CARTESIAN_POINT('',(27.5,-15.,2.02072594216369));
#32429=CARTESIAN_POINT('',(25.5,-15.,0.866025403784438));
#32430=CARTESIAN_POINT('',(27.5,-15.,2.02072594216369));
#32431=CARTESIAN_POINT('Origin',(27.75,-14.75,-0.866025403784439));
#32432=CARTESIAN_POINT('',(27.5,-15.,-0.866025403784439));
#32433=CARTESIAN_POINT('',(28.,-14.5,-0.866025403784439));
#32434=CARTESIAN_POINT('Origin',(23.,-15.,0.));
#32435=CARTESIAN_POINT('',(30.5,-15.,9.5));
#32436=CARTESIAN_POINT('',(22.1377898454666,-15.,-2.68587995320559));
#32437=CARTESIAN_POINT('',(21.7858117520809,-15.,-2.59788546711206));
#32438=CARTESIAN_POINT('Ctrl Pts',(22.1377898454666,-15.,-2.68587995320559));
#32439=CARTESIAN_POINT('Ctrl Pts',(21.9311050772667,-15.,-2.6388131454587));
#32440=CARTESIAN_POINT('Ctrl Pts',(21.7858117520809,-15.,-2.59788546711206));
#32441=CARTESIAN_POINT('',(19.5,-15.,-1.96145985275507));
#32442=CARTESIAN_POINT('',(22.0135911285113,-15.,-2.66130478825719));
#32443=CARTESIAN_POINT('',(19.5,-15.,-1.55627567321062));
#32444=CARTESIAN_POINT('',(19.5,-15.,-0.980729926377535));
#32445=CARTESIAN_POINT('',(22.5000001192093,-15.,-0.760232009924948));
#32446=CARTESIAN_POINT('',(21.3277838813459,-15.,-1.07127710028236));
#32447=CARTESIAN_POINT('',(22.5000001192093,-15.,-1.16746257990599));
#32448=CARTESIAN_POINT('',(22.5000001192093,-15.,-0.380116004962474));
#32449=CARTESIAN_POINT('',(20.5334244370461,-15.,-1.62380639463663));
#32450=CARTESIAN_POINT('',(22.8657597569362,-15.,-1.08258806942125));
#32451=CARTESIAN_POINT('',(19.9195088148117,-15.,-1.75068225711584));
#32452=CARTESIAN_POINT('Ctrl Pts',(20.5334244370461,-15.,-1.62380639463663));
#32453=CARTESIAN_POINT('Ctrl Pts',(20.2244202494621,-15.,-1.69747624546289));
#32454=CARTESIAN_POINT('Ctrl Pts',(19.9195088148117,-15.,-1.75068225711584));
#32455=CARTESIAN_POINT('',(20.4740790724754,-15.,-1.88574362546206));
#32456=CARTESIAN_POINT('Ctrl Pts',(19.9195088148117,-15.,-1.75068225711584));
#32457=CARTESIAN_POINT('Ctrl Pts',(20.4004092216492,-15.,-1.86527978628874));
#32458=CARTESIAN_POINT('Ctrl Pts',(20.4740790724754,-15.,-1.88574362546206));
#32459=CARTESIAN_POINT('',(22.5000001192093,-15.,-2.45668489485979));
#32460=CARTESIAN_POINT('',(21.3979462915622,-15.,-2.14610615225978));
#32461=CARTESIAN_POINT('',(22.5000001192093,-15.,-2.9355389252305));
#32462=CARTESIAN_POINT('',(22.5000001192093,-15.,-1.2283424474299));
#32463=CARTESIAN_POINT('',(20.9815825223923,-15.,-3.36527977138758));
#32464=CARTESIAN_POINT('',(23.1160603005779,-15.,-2.7611822632819));
#32465=CARTESIAN_POINT('',(19.9195088148117,-15.,-3.59856758266687));
#32466=CARTESIAN_POINT('Ctrl Pts',(20.9815825223923,-15.,-3.36527977138758));
#32467=CARTESIAN_POINT('Ctrl Pts',(20.4167805314064,-15.,-3.52694425731897));
#32468=CARTESIAN_POINT('Ctrl Pts',(19.9195088148117,-15.,-3.59856758266687));
#32469=CARTESIAN_POINT('',(20.5723057389259,-15.,-3.74795380979776));
#32470=CARTESIAN_POINT('Ctrl Pts',(19.9195088148117,-15.,-3.59856758266687));
#32471=CARTESIAN_POINT('Ctrl Pts',(20.2039561867714,-15.,-3.65586642175913));
#32472=CARTESIAN_POINT('Ctrl Pts',(20.5723057389259,-15.,-3.74795380979776));
#32473=CARTESIAN_POINT('',(22.5000001192093,-15.,-4.21862218528986));
#32474=CARTESIAN_POINT('',(21.2860505117679,-15.,-3.92222266495732));
#32475=CARTESIAN_POINT('',(22.5000001192093,-15.,-4.61766723543406));
#32476=CARTESIAN_POINT('',(22.5000001192093,-15.,-2.10931109264493));
#32477=CARTESIAN_POINT('',(19.5,-15.,-3.79502061754465));
#32478=CARTESIAN_POINT('',(22.1436755540772,-15.,-4.51995750652441));
#32479=CARTESIAN_POINT('',(19.5,-15.,-3.41234657913446));
#32480=CARTESIAN_POINT('',(19.5,-15.,-1.89751030877233));
#32481=CARTESIAN_POINT('',(21.7858117520809,-15.,-2.78001371771097));
#32482=CARTESIAN_POINT('',(21.5640325293677,-15.,-2.84136535367788));
#32483=CARTESIAN_POINT('Ctrl Pts',(21.7858117520809,-15.,-2.78001371771097));
#32484=CARTESIAN_POINT('Ctrl Pts',(22.0723055005074,-15.,-2.70020473748446));
#32485=CARTESIAN_POINT('Ctrl Pts',(22.1377898454666,-15.,-2.68587995320559));
#32486=CARTESIAN_POINT('',(20.4085947275162,-15.,0.0992497429251671));
#32487=CARTESIAN_POINT('',(20.4085947275162,-15.,1.3536836579442));
#32488=CARTESIAN_POINT('',(20.4085947275162,-15.,0.0496248714625835));
#32489=CARTESIAN_POINT('',(19.5,-15.,1.68315164744854));
#32490=CARTESIAN_POINT('',(21.7706366750829,-15.,0.859789946594888));
#32491=CARTESIAN_POINT('',(19.5,-15.,2.10470690100919));
#32492=CARTESIAN_POINT('',(19.5,-15.,0.84157582372427));
#32493=CARTESIAN_POINT('',(22.5000001192093,-15.,0.952592231333256));
#32494=CARTESIAN_POINT('',(21.3772735898822,-15.,1.38376211569081));
#32495=CARTESIAN_POINT('',(22.5000001192093,-15.,0.524897836148739));
#32496=CARTESIAN_POINT('',(22.5000001192093,-15.,0.476296115666628));
#32497=CARTESIAN_POINT('',(19.5,-15.,-0.702932812273502));
#32498=CARTESIAN_POINT('',(22.6221283822359,-15.,0.574882108956754));
#32499=CARTESIAN_POINT('',(19.5,-15.,-0.250681973993778));
#32500=CARTESIAN_POINT('',(19.5,-15.,-0.351466406136751));
#32501=CARTESIAN_POINT('',(21.0659912340793,-15.,0.352436209092567));
#32502=CARTESIAN_POINT('',(19.6258525252342,-15.,3.89631662517786));
#32503=CARTESIAN_POINT('',(19.4488404393196,-15.,4.44167826324701));
#32504=CARTESIAN_POINT('Ctrl Pts',(19.6258525252342,-15.,3.89631662517786));
#32505=CARTESIAN_POINT('Ctrl Pts',(19.4488404393196,-15.,4.11221016198397));
#32506=CARTESIAN_POINT('Ctrl Pts',(19.4488404393196,-15.,4.44167826324701));
#32507=CARTESIAN_POINT('',(19.7598908543587,-15.,5.12312430888414));
#32508=CARTESIAN_POINT('Ctrl Pts',(19.4488404393196,-15.,4.44167826324701));
#32509=CARTESIAN_POINT('Ctrl Pts',(19.4488404393196,-15.,4.87551178783178));
#32510=CARTESIAN_POINT('Ctrl Pts',(19.7598908543587,-15.,5.12312430888414));
#32511=CARTESIAN_POINT('',(20.9795362949371,-15.,5.41985012590885));
#32512=CARTESIAN_POINT('Ctrl Pts',(19.7598908543587,-15.,5.12312430888414));
#32513=CARTESIAN_POINT('Ctrl Pts',(20.1343790888786,-15.,5.41985012590885));
#32514=CARTESIAN_POINT('Ctrl Pts',(20.9795362949371,-15.,5.41985012590885));
#32515=CARTESIAN_POINT('',(21.8359481990337,-15.,5.31036853790283));
#32516=CARTESIAN_POINT('Ctrl Pts',(20.9795362949371,-15.,5.41985012590885));
#32517=CARTESIAN_POINT('Ctrl Pts',(21.511596262455,-15.,5.41985012590885));
#32518=CARTESIAN_POINT('Ctrl Pts',(21.8359481990337,-15.,5.31036853790283));
#32519=CARTESIAN_POINT('',(22.3362894058228,-15.,4.9849933758378));
#32520=CARTESIAN_POINT('Ctrl Pts',(21.8359481990337,-15.,5.31036853790283));
#32521=CARTESIAN_POINT('Ctrl Pts',(22.1603001356125,-15.,5.20088694989681));
#32522=CARTESIAN_POINT('Ctrl Pts',(22.3362894058228,-15.,4.9849933758378));
#32523=CARTESIAN_POINT('',(22.5122783780098,-15.,4.44167826324701));
#32524=CARTESIAN_POINT('Ctrl Pts',(22.3362894058228,-15.,4.9849933758378));
#32525=CARTESIAN_POINT('Ctrl Pts',(22.5122783780098,-15.,4.7690998390317));
#32526=CARTESIAN_POINT('Ctrl Pts',(22.5122783780098,-15.,4.44167826324701));
#32527=CARTESIAN_POINT('',(22.4150751233101,-15.,4.01807654649019));
#32528=CARTESIAN_POINT('Ctrl Pts',(22.5122783780098,-15.,4.44167826324701));
#32529=CARTESIAN_POINT('Ctrl Pts',(22.5122783780098,-15.,4.2002047970891));
#32530=CARTESIAN_POINT('Ctrl Pts',(22.4150751233101,-15.,4.01807654649019));
#32531=CARTESIAN_POINT('',(22.1347205042839,-15.,3.71725801378489));
#32532=CARTESIAN_POINT('Ctrl Pts',(22.4150751233101,-15.,4.01807654649019));
#32533=CARTESIAN_POINT('Ctrl Pts',(22.3178718686104,-15.,3.83594829589128));
#32534=CARTESIAN_POINT('Ctrl Pts',(22.1347205042839,-15.,3.71725801378489));
#32535=CARTESIAN_POINT('',(21.6886084973812,-15.,3.53103701025248));
#32536=CARTESIAN_POINT('Ctrl Pts',(22.1347205042839,-15.,3.71725801378489));
#32537=CARTESIAN_POINT('Ctrl Pts',(21.9515691399574,-15.,3.59856758266687));
#32538=CARTESIAN_POINT('Ctrl Pts',(21.6886084973812,-15.,3.53103701025248));
#32539=CARTESIAN_POINT('',(20.9795362949371,-15.,3.46350628882647));
#32540=CARTESIAN_POINT('Ctrl Pts',(21.6886084973812,-15.,3.53103701025248));
#32541=CARTESIAN_POINT('Ctrl Pts',(21.4256481528282,-15.,3.46350628882647));
#32542=CARTESIAN_POINT('Ctrl Pts',(20.9795362949371,-15.,3.46350628882647));
#32543=CARTESIAN_POINT('',(20.1272169947624,-15.,3.57196468859911));
#32544=CARTESIAN_POINT('Ctrl Pts',(20.9795362949371,-15.,3.46350628882647));
#32545=CARTESIAN_POINT('Ctrl Pts',(20.4515687823296,-15.,3.46350628882647));
#32546=CARTESIAN_POINT('Ctrl Pts',(20.1272169947624,-15.,3.57196468859911));
#32547=CARTESIAN_POINT('Ctrl Pts',(20.1272169947624,-15.,3.57196468859911));
#32548=CARTESIAN_POINT('Ctrl Pts',(19.8028649091721,-15.,3.68042308837175));
#32549=CARTESIAN_POINT('Ctrl Pts',(19.6258525252342,-15.,3.89631662517786));
#32550=CARTESIAN_POINT('',(22.1111871004105,-15.,6.9280356541276));
#32551=CARTESIAN_POINT('',(22.5122783780098,-15.,6.60061407834291));
#32552=CARTESIAN_POINT('Ctrl Pts',(22.1111871004105,-15.,6.9280356541276));
#32553=CARTESIAN_POINT('Ctrl Pts',(22.3178718686104,-15.,6.69679414480925));
#32554=CARTESIAN_POINT('Ctrl Pts',(22.5122783780098,-15.,6.60061407834291));
#32555=CARTESIAN_POINT('',(22.5122783780098,-15.,6.3632333651185));
#32556=CARTESIAN_POINT('',(22.5122783780098,-15.,3.30030703917146));
#32557=CARTESIAN_POINT('',(19.5,-15.,6.3632333651185));
#32558=CARTESIAN_POINT('',(22.7561391890049,-15.,6.3632333651185));
#32559=CARTESIAN_POINT('',(19.5,-15.,6.73158269375563));
#32560=CARTESIAN_POINT('',(19.5,-15.,3.18161668255925));
#32561=CARTESIAN_POINT('',(21.8472033441067,-15.,6.73158269375563));
#32562=CARTESIAN_POINT('',(21.25,-15.,6.73158269375563));
#32563=CARTESIAN_POINT('',(21.5934516191483,-15.,7.080491296947));
#32564=CARTESIAN_POINT('Ctrl Pts',(21.8472033441067,-15.,6.73158269375563));
#32565=CARTESIAN_POINT('Ctrl Pts',(21.7203274071217,-15.,6.86459768563509));
#32566=CARTESIAN_POINT('Ctrl Pts',(21.5934516191483,-15.,7.080491296947));
#32567=CARTESIAN_POINT('',(21.4031378626823,-15.,7.46828120201826));
#32568=CARTESIAN_POINT('Ctrl Pts',(21.5934516191483,-15.,7.080491296947));
#32569=CARTESIAN_POINT('Ctrl Pts',(21.4665756821632,-15.,7.29638490825891));
#32570=CARTESIAN_POINT('Ctrl Pts',(21.4031378626823,-15.,7.46828120201826));
#32571=CARTESIAN_POINT('',(21.7592087090015,-15.,7.46828120201826));
#32572=CARTESIAN_POINT('',(22.2015689313412,-15.,7.46828120201826));
#32573=CARTESIAN_POINT('Ctrl Pts',(21.7592087090015,-15.,7.46828120201826));
#32574=CARTESIAN_POINT('Ctrl Pts',(21.9045020341873,-15.,7.15927708894014));
#32575=CARTESIAN_POINT('Ctrl Pts',(22.1111871004105,-15.,6.9280356541276));
#32576=CARTESIAN_POINT('',(19.9062074422836,-15.,-6.90143261104822));
#32577=CARTESIAN_POINT('',(20.1180080771446,-15.,-7.27387461811304));
#32578=CARTESIAN_POINT('Ctrl Pts',(19.9062074422836,-15.,-6.90143261104822));
#32579=CARTESIAN_POINT('Ctrl Pts',(20.0054569244385,-15.,-7.14699868112802));
#32580=CARTESIAN_POINT('Ctrl Pts',(20.1180080771446,-15.,-7.27387461811304));
#32581=CARTESIAN_POINT('',(20.6766710877419,-15.,-7.27387461811304));
#32582=CARTESIAN_POINT('',(21.5590040385723,-15.,-7.27387461811304));
#32583=CARTESIAN_POINT('',(20.6766710877419,-15.,-6.39188278466463));
#32584=CARTESIAN_POINT('',(20.6766710877419,-15.,-3.63693730905652));
#32585=CARTESIAN_POINT('',(21.0286494791508,-15.,-6.39188278466463));
#32586=CARTESIAN_POINT('',(21.8383355438709,-15.,-6.39188278466463));
#32587=CARTESIAN_POINT('',(21.0306958556175,-15.,-7.66268793493509));
#32588=CARTESIAN_POINT('',(21.0235056266662,-15.,-3.19753690751813));
#32589=CARTESIAN_POINT('',(19.9174625873566,-15.,-7.66268793493509));
#32590=CARTESIAN_POINT('',(22.0153479278088,-15.,-7.66268793493509));
#32591=CARTESIAN_POINT('',(19.5665074586868,-15.,-7.0590041950345));
#32592=CARTESIAN_POINT('Ctrl Pts',(19.9174625873566,-15.,-7.66268793493509));
#32593=CARTESIAN_POINT('Ctrl Pts',(19.684174478054,-15.,-7.37005475908518));
#32594=CARTESIAN_POINT('Ctrl Pts',(19.5665074586868,-15.,-7.0590041950345));
#32595=CARTESIAN_POINT('',(19.4488404393196,-15.,-6.42053220421076));
#32596=CARTESIAN_POINT('Ctrl Pts',(19.5665074586868,-15.,-7.0590041950345));
#32597=CARTESIAN_POINT('Ctrl Pts',(19.4488404393196,-15.,-6.74795377999544));
#32598=CARTESIAN_POINT('Ctrl Pts',(19.4488404393196,-15.,-6.42053220421076));
#32599=CARTESIAN_POINT('',(19.638131082058,-15.,-5.61732616275549));
#32600=CARTESIAN_POINT('Ctrl Pts',(19.4488404393196,-15.,-6.42053220421076));
#32601=CARTESIAN_POINT('Ctrl Pts',(19.4488404393196,-15.,-5.97851309925318));
#32602=CARTESIAN_POINT('Ctrl Pts',(19.638131082058,-15.,-5.61732616275549));
#32603=CARTESIAN_POINT('',(20.1855389475822,-15.,-5.07196459919214));
#32604=CARTESIAN_POINT('Ctrl Pts',(19.638131082058,-15.,-5.61732616275549));
#32605=CARTESIAN_POINT('Ctrl Pts',(19.8274214267731,-15.,-5.2561392262578));
#32606=CARTESIAN_POINT('Ctrl Pts',(20.1855389475822,-15.,-5.07196459919214));
#32607=CARTESIAN_POINT('',(20.9856754243374,-15.,-4.88778999075293));
#32608=CARTESIAN_POINT('Ctrl Pts',(20.1855389475822,-15.,-5.07196459919214));
#32609=CARTESIAN_POINT('Ctrl Pts',(20.5436561703682,-15.,-4.88778999075293));
#32610=CARTESIAN_POINT('Ctrl Pts',(20.9856754243374,-15.,-4.88778999075293));
#32611=CARTESIAN_POINT('',(21.8032061755657,-15.,-5.07094141095877));
#32612=CARTESIAN_POINT('Ctrl Pts',(20.9856754243374,-15.,-4.88778999075293));
#32613=CARTESIAN_POINT('Ctrl Pts',(21.4236017763615,-15.,-4.88778999075293));
#32614=CARTESIAN_POINT('Ctrl Pts',(21.8032061755657,-15.,-5.07094141095877));
#32615=CARTESIAN_POINT('',(22.3669852018356,-15.,-5.59788551181555));
#32616=CARTESIAN_POINT('Ctrl Pts',(21.8032061755657,-15.,-5.07094141095877));
#32617=CARTESIAN_POINT('Ctrl Pts',(22.1828104257584,-15.,-5.25409284979105));
#32618=CARTESIAN_POINT('Ctrl Pts',(22.3669852018356,-15.,-5.59788551181555));
#32619=CARTESIAN_POINT('',(22.5511596798897,-15.,-6.38983640819788));
#32620=CARTESIAN_POINT('Ctrl Pts',(22.3669852018356,-15.,-5.59788551181555));
#32621=CARTESIAN_POINT('Ctrl Pts',(22.5511596798897,-15.,-5.94167817384004));
#32622=CARTESIAN_POINT('Ctrl Pts',(22.5511596798897,-15.,-6.38983640819788));
#32623=CARTESIAN_POINT('',(22.445770919323,-15.,-6.9781719520688));
#32624=CARTESIAN_POINT('Ctrl Pts',(22.5511596798897,-15.,-6.38983640819788));
#32625=CARTESIAN_POINT('Ctrl Pts',(22.5511596798897,-15.,-6.71521160751581));
#32626=CARTESIAN_POINT('Ctrl Pts',(22.445770919323,-15.,-6.9781719520688));
#32627=CARTESIAN_POINT('',(22.1521146297455,-15.,-7.39051882177591));
#32628=CARTESIAN_POINT('Ctrl Pts',(22.445770919323,-15.,-6.9781719520688));
#32629=CARTESIAN_POINT('Ctrl Pts',(22.3403821587563,-15.,-7.24113259464502));
#32630=CARTESIAN_POINT('Ctrl Pts',(22.1521146297455,-15.,-7.39051882177591));
#32631=CARTESIAN_POINT('',(21.6609823405743,-15.,-7.61766735464334));
#32632=CARTESIAN_POINT('Ctrl Pts',(22.1521146297455,-15.,-7.39051882177591));
#32633=CARTESIAN_POINT('Ctrl Pts',(21.9638473987579,-15.,-7.53990475088358));
#32634=CARTESIAN_POINT('Ctrl Pts',(21.6609823405743,-15.,-7.61766735464334));
#32635=CARTESIAN_POINT('',(21.562755972147,-15.,-7.25955013185739));
#32636=CARTESIAN_POINT('',(20.7362158118188,-15.,-4.2461203219493));
#32637=CARTESIAN_POINT('',(21.9229195713997,-15.,-7.09174636751413));
#32638=CARTESIAN_POINT('Ctrl Pts',(21.562755972147,-15.,-7.25955013185739));
#32639=CARTESIAN_POINT('Ctrl Pts',(21.7919510304928,-15.,-7.19201926141977));
#32640=CARTESIAN_POINT('Ctrl Pts',(21.9229195713997,-15.,-7.09174636751413));
#32641=CARTESIAN_POINT('',(22.1326739788055,-15.,-6.80525247007608));
#32642=CARTESIAN_POINT('Ctrl Pts',(21.9229195713997,-15.,-7.09174636751413));
#32643=CARTESIAN_POINT('Ctrl Pts',(22.0538882613182,-15.,-6.99147347360849));
#32644=CARTESIAN_POINT('Ctrl Pts',(22.1326739788055,-15.,-6.80525247007608));
#32645=CARTESIAN_POINT('',(22.2114599943161,-15.,-6.39188278466463));
#32646=CARTESIAN_POINT('Ctrl Pts',(22.1326739788055,-15.,-6.80525247007608));
#32647=CARTESIAN_POINT('Ctrl Pts',(22.2114599943161,-15.,-6.61903146654367));
#32648=CARTESIAN_POINT('Ctrl Pts',(22.2114599943161,-15.,-6.39188278466463));
#32649=CARTESIAN_POINT('',(22.128581225872,-15.,-5.92121426016092));
#32650=CARTESIAN_POINT('Ctrl Pts',(22.2114599943161,-15.,-6.39188278466463));
#32651=CARTESIAN_POINT('Ctrl Pts',(22.2114599943161,-15.,-6.11971367150545));
#32652=CARTESIAN_POINT('Ctrl Pts',(22.128581225872,-15.,-5.92121426016092));
#32653=CARTESIAN_POINT('',(21.9106413125992,-15.,-5.60095507651567));
#32654=CARTESIAN_POINT('Ctrl Pts',(22.128581225872,-15.,-5.92121426016092));
#32655=CARTESIAN_POINT('Ctrl Pts',(22.0457027554512,-15.,-5.7227149233222));
#32656=CARTESIAN_POINT('Ctrl Pts',(21.9106413125992,-15.,-5.60095507651567));
#32657=CARTESIAN_POINT('',(21.6139155328274,-15.,-5.41166450828314));
#32658=CARTESIAN_POINT('Ctrl Pts',(21.9106413125992,-15.,-5.60095507651567));
#32659=CARTESIAN_POINT('Ctrl Pts',(21.7755798697472,-15.,-5.47919515520334));
#32660=CARTESIAN_POINT('Ctrl Pts',(21.6139155328274,-15.,-5.41166450828314));
#32661=CARTESIAN_POINT('',(21.0102319419384,-15.,-5.29706697911024));
#32662=CARTESIAN_POINT('Ctrl Pts',(21.6139155328274,-15.,-5.41166450828314));
#32663=CARTESIAN_POINT('Ctrl Pts',(21.3356071412563,-15.,-5.29706697911024));
#32664=CARTESIAN_POINT('Ctrl Pts',(21.0102319419384,-15.,-5.29706697911024));
#32665=CARTESIAN_POINT('',(20.3390176296234,-15.,-5.43519791215658));
#32666=CARTESIAN_POINT('Ctrl Pts',(21.0102319419384,-15.,-5.29706697911024));
#32667=CARTESIAN_POINT('Ctrl Pts',(20.6091405153275,-15.,-5.29706697911024));
#32668=CARTESIAN_POINT('Ctrl Pts',(20.3390176296234,-15.,-5.43519791215658));
#32669=CARTESIAN_POINT('',(19.9379263520241,-15.,-5.8373125270009));
#32670=CARTESIAN_POINT('Ctrl Pts',(20.3390176296234,-15.,-5.43519791215658));
#32671=CARTESIAN_POINT('Ctrl Pts',(20.0688950419426,-15.,-5.57332884520292));
#32672=CARTESIAN_POINT('Ctrl Pts',(19.9379263520241,-15.,-5.8373125270009));
#32673=CARTESIAN_POINT('',(19.8069576621056,-15.,-6.39802191406488));
#32674=CARTESIAN_POINT('Ctrl Pts',(19.9379263520241,-15.,-5.8373125270009));
#32675=CARTESIAN_POINT('Ctrl Pts',(19.8069576621056,-15.,-6.10129613429308));
#32676=CARTESIAN_POINT('Ctrl Pts',(19.8069576621056,-15.,-6.39802191406488));
#32677=CARTESIAN_POINT('Ctrl Pts',(19.8069576621056,-15.,-6.39802191406488));
#32678=CARTESIAN_POINT('Ctrl Pts',(19.8069576621056,-15.,-6.6558663919568));
#32679=CARTESIAN_POINT('Ctrl Pts',(19.9062074422836,-15.,-6.90143261104822));
#32680=CARTESIAN_POINT('Origin',(30.75,-14.75,9.5));
#32681=CARTESIAN_POINT('',(31.,-14.5,3.96410161513775));
#32682=CARTESIAN_POINT('',(31.7722431864335,-13.7277568135665,5.30166604983953));
#32683=CARTESIAN_POINT('',(31.,-14.5,17.5));
#32684=CARTESIAN_POINT('',(31.,-14.5,9.5));
#32685=CARTESIAN_POINT('',(30.6464466094067,-14.8535533905933,18.3535533905933));
#32686=CARTESIAN_POINT('',(32.0925950670041,-13.4074049329959,14.8622421710567));
#32687=CARTESIAN_POINT('',(32.0833333333333,-13.4166666666667,16.9166666666667));
#32688=CARTESIAN_POINT('Origin',(30.7834936490539,-15.,3.58910161513775));
#32689=CARTESIAN_POINT('',(31.,-15.,3.96410161513775));
#32690=CARTESIAN_POINT('',(30.5669872981078,-15.,3.21410161513775));
#32691=CARTESIAN_POINT('Origin',(31.,-15.,19.));
#32692=CARTESIAN_POINT('',(31.,-15.,17.5));
#32693=CARTESIAN_POINT('Origin',(29.9267766952966,-15.,18.8232233047034));
#32694=CARTESIAN_POINT('',(30.3535533905933,14.8535533905933,18.6464466094067));
#32695=CARTESIAN_POINT('',(30.3535533905933,-15.,18.6464466094067));
#32696=CARTESIAN_POINT('',(21.3057316934887,11.105822933719,22.394177066281));
#32697=CARTESIAN_POINT('Origin',(19.,14.75,18.75));
#32698=CARTESIAN_POINT('',(23.5,8.00000000000003,25.5));
#32699=CARTESIAN_POINT('',(21.1666666666667,9.33333333333336,24.1666666666667));
#32700=CARTESIAN_POINT('Origin',(30.5,-15.,18.5));
#32701=CARTESIAN_POINT('',(30.6464466094067,-15.,18.3535533905933));
#32702=CARTESIAN_POINT('Origin',(30.8232233047034,-15.,17.9267766952966));
#32703=CARTESIAN_POINT('Ctrl Pts',(22.1377898454666,-15.,-2.68587995320559));
#32704=CARTESIAN_POINT('Ctrl Pts',(22.1377898454666,-14.75,-2.68587995320559));
#32705=CARTESIAN_POINT('Ctrl Pts',(21.9311050772667,-15.,-2.6388131454587));
#32706=CARTESIAN_POINT('Ctrl Pts',(21.9311050772667,-14.75,-2.6388131454587));
#32707=CARTESIAN_POINT('Ctrl Pts',(21.7858117520809,-15.,-2.59788546711206));
#32708=CARTESIAN_POINT('Ctrl Pts',(21.7858117520809,-14.75,-2.59788546711206));
#32709=CARTESIAN_POINT('',(22.1377898454666,-14.75,-2.68587995320559));
#32710=CARTESIAN_POINT('',(22.1377898454666,-15.,-2.68587995320559));
#32711=CARTESIAN_POINT('',(21.7858117520809,-14.75,-2.59788546711206));
#32712=CARTESIAN_POINT('Ctrl Pts',(22.1377898454666,-14.75,-2.68587995320559));
#32713=CARTESIAN_POINT('Ctrl Pts',(21.9311050772667,-14.75,-2.6388131454587));
#32714=CARTESIAN_POINT('Ctrl Pts',(21.7858117520809,-14.75,-2.59788546711206));
#32715=CARTESIAN_POINT('',(21.7858117520809,-15.,-2.59788546711206));
#32716=CARTESIAN_POINT('Ctrl Pts',(21.7858117520809,-15.,-2.78001371771097));
#32717=CARTESIAN_POINT('Ctrl Pts',(21.7858117520809,-14.75,-2.78001371771097));
#32718=CARTESIAN_POINT('Ctrl Pts',(22.0723055005074,-15.,-2.70020473748446));
#32719=CARTESIAN_POINT('Ctrl Pts',(22.0723055005074,-14.75,-2.70020473748446));
#32720=CARTESIAN_POINT('Ctrl Pts',(22.1377898454666,-15.,-2.68587995320559));
#32721=CARTESIAN_POINT('Ctrl Pts',(22.1377898454666,-14.75,-2.68587995320559));
#32722=CARTESIAN_POINT('',(21.7858117520809,-14.75,-2.78001371771097));
#32723=CARTESIAN_POINT('',(21.7858117520809,-15.,-2.78001371771097));
#32724=CARTESIAN_POINT('Ctrl Pts',(21.7858117520809,-14.75,-2.78001371771097));
#32725=CARTESIAN_POINT('Ctrl Pts',(22.0723055005074,-14.75,-2.70020473748446));
#32726=CARTESIAN_POINT('Ctrl Pts',(22.1377898454666,-14.75,-2.68587995320559));
#32727=CARTESIAN_POINT('Origin',(19.5,-15.,-3.41234657913446));
#32728=CARTESIAN_POINT('',(19.5,-14.75,-3.41234657913446));
#32729=CARTESIAN_POINT('',(19.5,-15.,-3.41234657913446));
#32730=CARTESIAN_POINT('',(19.5,-14.75,-3.41234657913446));
#32731=CARTESIAN_POINT('Origin',(19.5,-15.,-3.79502061754465));
#32732=CARTESIAN_POINT('',(19.5,-14.75,-3.79502061754465));
#32733=CARTESIAN_POINT('',(19.5,-15.,-3.79502061754465));
#32734=CARTESIAN_POINT('',(19.5,-14.75,-3.79502061754465));
#32735=CARTESIAN_POINT('Origin',(22.5000001192093,-15.,-4.61766723543406));
#32736=CARTESIAN_POINT('',(22.5000001192093,-14.75,-4.61766723543406));
#32737=CARTESIAN_POINT('',(22.5000001192093,-15.,-4.61766723543406));
#32738=CARTESIAN_POINT('',(22.5000001192093,-14.75,-4.61766723543406));
#32739=CARTESIAN_POINT('Origin',(22.5000001192093,-15.,-4.21862218528986));
#32740=CARTESIAN_POINT('',(22.5000001192093,-14.75,-4.21862218528986));
#32741=CARTESIAN_POINT('',(22.5000001192093,-15.,-4.21862218528986));
#32742=CARTESIAN_POINT('',(22.5000001192093,-14.75,-4.21862218528986));
#32743=CARTESIAN_POINT('Origin',(20.5723057389259,-15.,-3.74795380979776));
#32744=CARTESIAN_POINT('',(20.5723057389259,-14.75,-3.74795380979776));
#32745=CARTESIAN_POINT('',(20.5723057389259,-15.,-3.74795380979776));
#32746=CARTESIAN_POINT('',(20.5723057389259,-14.75,-3.74795380979776));
#32747=CARTESIAN_POINT('Ctrl Pts',(19.9195088148117,-15.,-3.59856758266687));
#32748=CARTESIAN_POINT('Ctrl Pts',(19.9195088148117,-14.75,-3.59856758266687));
#32749=CARTESIAN_POINT('Ctrl Pts',(20.2039561867714,-15.,-3.65586642175913));
#32750=CARTESIAN_POINT('Ctrl Pts',(20.2039561867714,-14.75,-3.65586642175913));
#32751=CARTESIAN_POINT('Ctrl Pts',(20.5723057389259,-15.,-3.74795380979776));
#32752=CARTESIAN_POINT('Ctrl Pts',(20.5723057389259,-14.75,-3.74795380979776));
#32753=CARTESIAN_POINT('',(19.9195088148117,-14.75,-3.59856758266687));
#32754=CARTESIAN_POINT('',(19.9195088148117,-15.,-3.59856758266687));
#32755=CARTESIAN_POINT('Ctrl Pts',(19.9195088148117,-14.75,-3.59856758266687));
#32756=CARTESIAN_POINT('Ctrl Pts',(20.2039561867714,-14.75,-3.65586642175913));
#32757=CARTESIAN_POINT('Ctrl Pts',(20.5723057389259,-14.75,-3.74795380979776));
#32758=CARTESIAN_POINT('Ctrl Pts',(20.9815825223923,-15.,-3.36527977138758));
#32759=CARTESIAN_POINT('Ctrl Pts',(20.9815825223923,-14.75,-3.36527977138758));
#32760=CARTESIAN_POINT('Ctrl Pts',(20.4167805314064,-15.,-3.52694425731897));
#32761=CARTESIAN_POINT('Ctrl Pts',(20.4167805314064,-14.75,-3.52694425731897));
#32762=CARTESIAN_POINT('Ctrl Pts',(19.9195088148117,-15.,-3.59856758266687));
#32763=CARTESIAN_POINT('Ctrl Pts',(19.9195088148117,-14.75,-3.59856758266687));
#32764=CARTESIAN_POINT('',(20.9815825223923,-14.75,-3.36527977138758));
#32765=CARTESIAN_POINT('',(20.9815825223923,-15.,-3.36527977138758));
#32766=CARTESIAN_POINT('Ctrl Pts',(20.9815825223923,-14.75,-3.36527977138758));
#32767=CARTESIAN_POINT('Ctrl Pts',(20.4167805314064,-14.75,-3.52694425731897));
#32768=CARTESIAN_POINT('Ctrl Pts',(19.9195088148117,-14.75,-3.59856758266687));
#32769=CARTESIAN_POINT('Origin',(22.5000001192093,-15.,-2.9355389252305));
#32770=CARTESIAN_POINT('',(22.5000001192093,-14.75,-2.9355389252305));
#32771=CARTESIAN_POINT('',(22.5000001192093,-15.,-2.9355389252305));
#32772=CARTESIAN_POINT('',(22.5000001192093,-14.75,-2.9355389252305));
#32773=CARTESIAN_POINT('Origin',(22.5000001192093,-15.,-2.45668489485979));
#32774=CARTESIAN_POINT('',(22.5000001192093,-14.75,-2.45668489485979));
#32775=CARTESIAN_POINT('',(22.5000001192093,-15.,-2.45668489485979));
#32776=CARTESIAN_POINT('',(22.5000001192093,-14.75,-2.45668489485979));
#32777=CARTESIAN_POINT('Origin',(20.4740790724754,-15.,-1.88574362546206));
#32778=CARTESIAN_POINT('',(20.4740790724754,-14.75,-1.88574362546206));
#32779=CARTESIAN_POINT('',(20.4740790724754,-15.,-1.88574362546206));
#32780=CARTESIAN_POINT('',(20.4740790724754,-14.75,-1.88574362546206));
#32781=CARTESIAN_POINT('Ctrl Pts',(19.9195088148117,-15.,-1.75068225711584));
#32782=CARTESIAN_POINT('Ctrl Pts',(19.9195088148117,-14.75,-1.75068225711584));
#32783=CARTESIAN_POINT('Ctrl Pts',(20.4004092216492,-15.,-1.86527978628874));
#32784=CARTESIAN_POINT('Ctrl Pts',(20.4004092216492,-14.75,-1.86527978628874));
#32785=CARTESIAN_POINT('Ctrl Pts',(20.4740790724754,-15.,-1.88574362546206));
#32786=CARTESIAN_POINT('Ctrl Pts',(20.4740790724754,-14.75,-1.88574362546206));
#32787=CARTESIAN_POINT('',(19.9195088148117,-14.75,-1.75068225711584));
#32788=CARTESIAN_POINT('',(19.9195088148117,-15.,-1.75068225711584));
#32789=CARTESIAN_POINT('Ctrl Pts',(19.9195088148117,-14.75,-1.75068225711584));
#32790=CARTESIAN_POINT('Ctrl Pts',(20.4004092216492,-14.75,-1.86527978628874));
#32791=CARTESIAN_POINT('Ctrl Pts',(20.4740790724754,-14.75,-1.88574362546206));
#32792=CARTESIAN_POINT('Ctrl Pts',(20.5334244370461,-15.,-1.62380639463663));
#32793=CARTESIAN_POINT('Ctrl Pts',(20.5334244370461,-14.75,-1.62380639463663));
#32794=CARTESIAN_POINT('Ctrl Pts',(20.2244202494621,-15.,-1.69747624546289));
#32795=CARTESIAN_POINT('Ctrl Pts',(20.2244202494621,-14.75,-1.69747624546289));
#32796=CARTESIAN_POINT('Ctrl Pts',(19.9195088148117,-15.,-1.75068225711584));
#32797=CARTESIAN_POINT('Ctrl Pts',(19.9195088148117,-14.75,-1.75068225711584));
#32798=CARTESIAN_POINT('',(20.5334244370461,-14.75,-1.62380639463663));
#32799=CARTESIAN_POINT('',(20.5334244370461,-15.,-1.62380639463663));
#32800=CARTESIAN_POINT('Ctrl Pts',(20.5334244370461,-14.75,-1.62380639463663));
#32801=CARTESIAN_POINT('Ctrl Pts',(20.2244202494621,-14.75,-1.69747624546289));
#32802=CARTESIAN_POINT('Ctrl Pts',(19.9195088148117,-14.75,-1.75068225711584));
#32803=CARTESIAN_POINT('Origin',(22.5000001192093,-15.,-1.16746257990599));
#32804=CARTESIAN_POINT('',(22.5000001192093,-14.75,-1.16746257990599));
#32805=CARTESIAN_POINT('',(22.5000001192093,-15.,-1.16746257990599));
#32806=CARTESIAN_POINT('',(22.5000001192093,-14.75,-1.16746257990599));
#32807=CARTESIAN_POINT('Origin',(22.5000001192093,-15.,-0.760232009924948));
#32808=CARTESIAN_POINT('',(22.5000001192093,-14.75,-0.760232009924948));
#32809=CARTESIAN_POINT('',(22.5000001192093,-15.,-0.760232009924948));
#32810=CARTESIAN_POINT('',(22.5000001192093,-14.75,-0.760232009924948));
#32811=CARTESIAN_POINT('Origin',(19.5,-15.,-1.55627567321062));
#32812=CARTESIAN_POINT('',(19.5,-14.75,-1.55627567321062));
#32813=CARTESIAN_POINT('',(19.5,-15.,-1.55627567321062));
#32814=CARTESIAN_POINT('',(19.5,-14.75,-1.55627567321062));
#32815=CARTESIAN_POINT('Origin',(19.5,-15.,-1.96145985275507));
#32816=CARTESIAN_POINT('',(19.5,-14.75,-1.96145985275507));
#32817=CARTESIAN_POINT('',(19.5,-15.,-1.96145985275507));
#32818=CARTESIAN_POINT('',(19.5,-14.75,-1.96145985275507));
#32819=CARTESIAN_POINT('Origin',(21.7858117520809,-15.,-2.59788546711206));
#32820=CARTESIAN_POINT('',(21.7858117520809,-14.75,-2.59788546711206));
#32821=CARTESIAN_POINT('Origin',(21.0000000596046,-14.75,-2.6889496226795));
#32822=CARTESIAN_POINT('Origin',(20.4085947275162,-15.,0.0992497429251671));
#32823=CARTESIAN_POINT('',(20.4085947275162,-14.75,0.0992497429251671));
#32824=CARTESIAN_POINT('',(20.4085947275162,-15.,0.0992497429251671));
#32825=CARTESIAN_POINT('',(20.4085947275162,-14.75,1.3536836579442));
#32826=CARTESIAN_POINT('',(20.4085947275162,-14.75,0.0992497429251671));
#32827=CARTESIAN_POINT('',(20.4085947275162,-15.,1.3536836579442));
#32828=CARTESIAN_POINT('Origin',(19.5,-15.,-0.250681973993778));
#32829=CARTESIAN_POINT('',(19.5,-14.75,-0.250681973993778));
#32830=CARTESIAN_POINT('',(19.5,-15.,-0.250681973993778));
#32831=CARTESIAN_POINT('',(19.5,-14.75,-0.250681973993778));
#32832=CARTESIAN_POINT('Origin',(19.5,-15.,-0.702932812273502));
#32833=CARTESIAN_POINT('',(19.5,-14.75,-0.702932812273502));
#32834=CARTESIAN_POINT('',(19.5,-15.,-0.702932812273502));
#32835=CARTESIAN_POINT('',(19.5,-14.75,-0.702932812273502));
#32836=CARTESIAN_POINT('Origin',(22.5000001192093,-15.,0.524897836148739));
#32837=CARTESIAN_POINT('',(22.5000001192093,-14.75,0.524897836148739));
#32838=CARTESIAN_POINT('',(22.5000001192093,-15.,0.524897836148739));
#32839=CARTESIAN_POINT('',(22.5000001192093,-14.75,0.524897836148739));
#32840=CARTESIAN_POINT('Origin',(22.5000001192093,-15.,0.952592231333256));
#32841=CARTESIAN_POINT('',(22.5000001192093,-14.75,0.952592231333256));
#32842=CARTESIAN_POINT('',(22.5000001192093,-15.,0.952592231333256));
#32843=CARTESIAN_POINT('',(22.5000001192093,-14.75,0.952592231333256));
#32844=CARTESIAN_POINT('Origin',(19.5,-15.,2.10470690100919));
#32845=CARTESIAN_POINT('',(19.5,-14.75,2.10470690100919));
#32846=CARTESIAN_POINT('',(19.5,-15.,2.10470690100919));
#32847=CARTESIAN_POINT('',(19.5,-14.75,2.10470690100919));
#32848=CARTESIAN_POINT('Origin',(19.5,-15.,1.68315164744854));
#32849=CARTESIAN_POINT('',(19.5,-14.75,1.68315164744854));
#32850=CARTESIAN_POINT('',(19.5,-15.,1.68315164744854));
#32851=CARTESIAN_POINT('',(19.5,-14.75,1.68315164744854));
#32852=CARTESIAN_POINT('Origin',(20.4085947275162,-15.,1.3536836579442));
#32853=CARTESIAN_POINT('',(20.4085947275162,-14.75,1.3536836579442));
#32854=CARTESIAN_POINT('Origin',(21.0000000596046,-14.75,0.700887044367846));
#32855=CARTESIAN_POINT('Ctrl Pts',(19.6258525252342,-15.,3.89631662517786));
#32856=CARTESIAN_POINT('Ctrl Pts',(19.6258525252342,-14.75,3.89631662517786));
#32857=CARTESIAN_POINT('Ctrl Pts',(19.4488404393196,-15.,4.11221016198397));
#32858=CARTESIAN_POINT('Ctrl Pts',(19.4488404393196,-14.75,4.11221016198397));
#32859=CARTESIAN_POINT('Ctrl Pts',(19.4488404393196,-15.,4.44167826324701));
#32860=CARTESIAN_POINT('Ctrl Pts',(19.4488404393196,-14.75,4.44167826324701));
#32861=CARTESIAN_POINT('',(19.6258525252342,-14.75,3.89631662517786));
#32862=CARTESIAN_POINT('',(19.6258525252342,-15.,3.89631662517786));
#32863=CARTESIAN_POINT('',(19.4488404393196,-14.75,4.44167826324701));
#32864=CARTESIAN_POINT('Ctrl Pts',(19.6258525252342,-14.75,3.89631662517786));
#32865=CARTESIAN_POINT('Ctrl Pts',(19.4488404393196,-14.75,4.11221016198397));
#32866=CARTESIAN_POINT('Ctrl Pts',(19.4488404393196,-14.75,4.44167826324701));
#32867=CARTESIAN_POINT('',(19.4488404393196,-15.,4.44167826324701));
#32868=CARTESIAN_POINT('Ctrl Pts',(20.1272169947624,-15.,3.57196468859911));
#32869=CARTESIAN_POINT('Ctrl Pts',(20.1272169947624,-14.75,3.57196468859911));
#32870=CARTESIAN_POINT('Ctrl Pts',(19.8028649091721,-15.,3.68042308837175));
#32871=CARTESIAN_POINT('Ctrl Pts',(19.8028649091721,-14.75,3.68042308837175));
#32872=CARTESIAN_POINT('Ctrl Pts',(19.6258525252342,-15.,3.89631662517786));
#32873=CARTESIAN_POINT('Ctrl Pts',(19.6258525252342,-14.75,3.89631662517786));
#32874=CARTESIAN_POINT('',(20.1272169947624,-14.75,3.57196468859911));
#32875=CARTESIAN_POINT('',(20.1272169947624,-15.,3.57196468859911));
#32876=CARTESIAN_POINT('Ctrl Pts',(20.1272169947624,-14.75,3.57196468859911));
#32877=CARTESIAN_POINT('Ctrl Pts',(19.8028649091721,-14.75,3.68042308837175));
#32878=CARTESIAN_POINT('Ctrl Pts',(19.6258525252342,-14.75,3.89631662517786));
#32879=CARTESIAN_POINT('Ctrl Pts',(20.9795362949371,-15.,3.46350628882647));
#32880=CARTESIAN_POINT('Ctrl Pts',(20.9795362949371,-14.75,3.46350628882647));
#32881=CARTESIAN_POINT('Ctrl Pts',(20.4515687823296,-15.,3.46350628882647));
#32882=CARTESIAN_POINT('Ctrl Pts',(20.4515687823296,-14.75,3.46350628882647));
#32883=CARTESIAN_POINT('Ctrl Pts',(20.1272169947624,-15.,3.57196468859911));
#32884=CARTESIAN_POINT('Ctrl Pts',(20.1272169947624,-14.75,3.57196468859911));
#32885=CARTESIAN_POINT('',(20.9795362949371,-14.75,3.46350628882647));
#32886=CARTESIAN_POINT('',(20.9795362949371,-15.,3.46350628882647));
#32887=CARTESIAN_POINT('Ctrl Pts',(20.9795362949371,-14.75,3.46350628882647));
#32888=CARTESIAN_POINT('Ctrl Pts',(20.4515687823296,-14.75,3.46350628882647));
#32889=CARTESIAN_POINT('Ctrl Pts',(20.1272169947624,-14.75,3.57196468859911));
#32890=CARTESIAN_POINT('Ctrl Pts',(21.6886084973812,-15.,3.53103701025248));
#32891=CARTESIAN_POINT('Ctrl Pts',(21.6886084973812,-14.75,3.53103701025248));
#32892=CARTESIAN_POINT('Ctrl Pts',(21.4256481528282,-15.,3.46350628882647));
#32893=CARTESIAN_POINT('Ctrl Pts',(21.4256481528282,-14.75,3.46350628882647));
#32894=CARTESIAN_POINT('Ctrl Pts',(20.9795362949371,-15.,3.46350628882647));
#32895=CARTESIAN_POINT('Ctrl Pts',(20.9795362949371,-14.75,3.46350628882647));
#32896=CARTESIAN_POINT('',(21.6886084973812,-14.75,3.53103701025248));
#32897=CARTESIAN_POINT('',(21.6886084973812,-15.,3.53103701025248));
#32898=CARTESIAN_POINT('Ctrl Pts',(21.6886084973812,-14.75,3.53103701025248));
#32899=CARTESIAN_POINT('Ctrl Pts',(21.4256481528282,-14.75,3.46350628882647));
#32900=CARTESIAN_POINT('Ctrl Pts',(20.9795362949371,-14.75,3.46350628882647));
#32901=CARTESIAN_POINT('Ctrl Pts',(22.1347205042839,-15.,3.71725801378489));
#32902=CARTESIAN_POINT('Ctrl Pts',(22.1347205042839,-14.75,3.71725801378489));
#32903=CARTESIAN_POINT('Ctrl Pts',(21.9515691399574,-15.,3.59856758266687));
#32904=CARTESIAN_POINT('Ctrl Pts',(21.9515691399574,-14.75,3.59856758266687));
#32905=CARTESIAN_POINT('Ctrl Pts',(21.6886084973812,-15.,3.53103701025248));
#32906=CARTESIAN_POINT('Ctrl Pts',(21.6886084973812,-14.75,3.53103701025248));
#32907=CARTESIAN_POINT('',(22.1347205042839,-14.75,3.71725801378489));
#32908=CARTESIAN_POINT('',(22.1347205042839,-15.,3.71725801378489));
#32909=CARTESIAN_POINT('Ctrl Pts',(22.1347205042839,-14.75,3.71725801378489));
#32910=CARTESIAN_POINT('Ctrl Pts',(21.9515691399574,-14.75,3.59856758266687));
#32911=CARTESIAN_POINT('Ctrl Pts',(21.6886084973812,-14.75,3.53103701025248));
#32912=CARTESIAN_POINT('Ctrl Pts',(22.4150751233101,-15.,4.01807654649019));
#32913=CARTESIAN_POINT('Ctrl Pts',(22.4150751233101,-14.75,4.01807654649019));
#32914=CARTESIAN_POINT('Ctrl Pts',(22.3178718686104,-15.,3.83594829589128));
#32915=CARTESIAN_POINT('Ctrl Pts',(22.3178718686104,-14.75,3.83594829589128));
#32916=CARTESIAN_POINT('Ctrl Pts',(22.1347205042839,-15.,3.71725801378489));
#32917=CARTESIAN_POINT('Ctrl Pts',(22.1347205042839,-14.75,3.71725801378489));
#32918=CARTESIAN_POINT('',(22.4150751233101,-14.75,4.01807654649019));
#32919=CARTESIAN_POINT('',(22.4150751233101,-15.,4.01807654649019));
#32920=CARTESIAN_POINT('Ctrl Pts',(22.4150751233101,-14.75,4.01807654649019));
#32921=CARTESIAN_POINT('Ctrl Pts',(22.3178718686104,-14.75,3.83594829589128));
#32922=CARTESIAN_POINT('Ctrl Pts',(22.1347205042839,-14.75,3.71725801378489));
#32923=CARTESIAN_POINT('Ctrl Pts',(22.5122783780098,-15.,4.44167826324701));
#32924=CARTESIAN_POINT('Ctrl Pts',(22.5122783780098,-14.75,4.44167826324701));
#32925=CARTESIAN_POINT('Ctrl Pts',(22.5122783780098,-15.,4.2002047970891));
#32926=CARTESIAN_POINT('Ctrl Pts',(22.5122783780098,-14.75,4.2002047970891));
#32927=CARTESIAN_POINT('Ctrl Pts',(22.4150751233101,-15.,4.01807654649019));
#32928=CARTESIAN_POINT('Ctrl Pts',(22.4150751233101,-14.75,4.01807654649019));
#32929=CARTESIAN_POINT('',(22.5122783780098,-14.75,4.44167826324701));
#32930=CARTESIAN_POINT('',(22.5122783780098,-15.,4.44167826324701));
#32931=CARTESIAN_POINT('Ctrl Pts',(22.5122783780098,-14.75,4.44167826324701));
#32932=CARTESIAN_POINT('Ctrl Pts',(22.5122783780098,-14.75,4.2002047970891));
#32933=CARTESIAN_POINT('Ctrl Pts',(22.4150751233101,-14.75,4.01807654649019));
#32934=CARTESIAN_POINT('Ctrl Pts',(22.3362894058228,-15.,4.9849933758378));
#32935=CARTESIAN_POINT('Ctrl Pts',(22.3362894058228,-14.75,4.9849933758378));
#32936=CARTESIAN_POINT('Ctrl Pts',(22.5122783780098,-15.,4.7690998390317));
#32937=CARTESIAN_POINT('Ctrl Pts',(22.5122783780098,-14.75,4.7690998390317));
#32938=CARTESIAN_POINT('Ctrl Pts',(22.5122783780098,-15.,4.44167826324701));
#32939=CARTESIAN_POINT('Ctrl Pts',(22.5122783780098,-14.75,4.44167826324701));
#32940=CARTESIAN_POINT('',(22.3362894058228,-14.75,4.9849933758378));
#32941=CARTESIAN_POINT('',(22.3362894058228,-15.,4.9849933758378));
#32942=CARTESIAN_POINT('Ctrl Pts',(22.3362894058228,-14.75,4.9849933758378));
#32943=CARTESIAN_POINT('Ctrl Pts',(22.5122783780098,-14.75,4.7690998390317));
#32944=CARTESIAN_POINT('Ctrl Pts',(22.5122783780098,-14.75,4.44167826324701));
#32945=CARTESIAN_POINT('Ctrl Pts',(21.8359481990337,-15.,5.31036853790283));
#32946=CARTESIAN_POINT('Ctrl Pts',(21.8359481990337,-14.75,5.31036853790283));
#32947=CARTESIAN_POINT('Ctrl Pts',(22.1603001356125,-15.,5.20088694989681));
#32948=CARTESIAN_POINT('Ctrl Pts',(22.1603001356125,-14.75,5.20088694989681));
#32949=CARTESIAN_POINT('Ctrl Pts',(22.3362894058228,-15.,4.9849933758378));
#32950=CARTESIAN_POINT('Ctrl Pts',(22.3362894058228,-14.75,4.9849933758378));
#32951=CARTESIAN_POINT('',(21.8359481990337,-14.75,5.31036853790283));
#32952=CARTESIAN_POINT('',(21.8359481990337,-15.,5.31036853790283));
#32953=CARTESIAN_POINT('Ctrl Pts',(21.8359481990337,-14.75,5.31036853790283));
#32954=CARTESIAN_POINT('Ctrl Pts',(22.1603001356125,-14.75,5.20088694989681));
#32955=CARTESIAN_POINT('Ctrl Pts',(22.3362894058228,-14.75,4.9849933758378));
#32956=CARTESIAN_POINT('Ctrl Pts',(20.9795362949371,-15.,5.41985012590885));
#32957=CARTESIAN_POINT('Ctrl Pts',(20.9795362949371,-14.75,5.41985012590885));
#32958=CARTESIAN_POINT('Ctrl Pts',(21.511596262455,-15.,5.41985012590885));
#32959=CARTESIAN_POINT('Ctrl Pts',(21.511596262455,-14.75,5.41985012590885));
#32960=CARTESIAN_POINT('Ctrl Pts',(21.8359481990337,-15.,5.31036853790283));
#32961=CARTESIAN_POINT('Ctrl Pts',(21.8359481990337,-14.75,5.31036853790283));
#32962=CARTESIAN_POINT('',(20.9795362949371,-14.75,5.41985012590885));
#32963=CARTESIAN_POINT('',(20.9795362949371,-15.,5.41985012590885));
#32964=CARTESIAN_POINT('Ctrl Pts',(20.9795362949371,-14.75,5.41985012590885));
#32965=CARTESIAN_POINT('Ctrl Pts',(21.511596262455,-14.75,5.41985012590885));
#32966=CARTESIAN_POINT('Ctrl Pts',(21.8359481990337,-14.75,5.31036853790283));
#32967=CARTESIAN_POINT('Ctrl Pts',(19.7598908543587,-15.,5.12312430888414));
#32968=CARTESIAN_POINT('Ctrl Pts',(19.7598908543587,-14.75,5.12312430888414));
#32969=CARTESIAN_POINT('Ctrl Pts',(20.1343790888786,-15.,5.41985012590885));
#32970=CARTESIAN_POINT('Ctrl Pts',(20.1343790888786,-14.75,5.41985012590885));
#32971=CARTESIAN_POINT('Ctrl Pts',(20.9795362949371,-15.,5.41985012590885));
#32972=CARTESIAN_POINT('Ctrl Pts',(20.9795362949371,-14.75,5.41985012590885));
#32973=CARTESIAN_POINT('',(19.7598908543587,-14.75,5.12312430888414));
#32974=CARTESIAN_POINT('',(19.7598908543587,-15.,5.12312430888414));
#32975=CARTESIAN_POINT('Ctrl Pts',(19.7598908543587,-14.75,5.12312430888414));
#32976=CARTESIAN_POINT('Ctrl Pts',(20.1343790888786,-14.75,5.41985012590885));
#32977=CARTESIAN_POINT('Ctrl Pts',(20.9795362949371,-14.75,5.41985012590885));
#32978=CARTESIAN_POINT('Ctrl Pts',(19.4488404393196,-15.,4.44167826324701));
#32979=CARTESIAN_POINT('Ctrl Pts',(19.4488404393196,-14.75,4.44167826324701));
#32980=CARTESIAN_POINT('Ctrl Pts',(19.4488404393196,-15.,4.87551178783178));
#32981=CARTESIAN_POINT('Ctrl Pts',(19.4488404393196,-14.75,4.87551178783178));
#32982=CARTESIAN_POINT('Ctrl Pts',(19.7598908543587,-15.,5.12312430888414));
#32983=CARTESIAN_POINT('Ctrl Pts',(19.7598908543587,-14.75,5.12312430888414));
#32984=CARTESIAN_POINT('Ctrl Pts',(19.4488404393196,-14.75,4.44167826324701));
#32985=CARTESIAN_POINT('Ctrl Pts',(19.4488404393196,-14.75,4.87551178783178));
#32986=CARTESIAN_POINT('Ctrl Pts',(19.7598908543587,-14.75,5.12312430888414));
#32987=CARTESIAN_POINT('Origin',(20.9805594086647,-14.75,4.44167820736766));
#32988=CARTESIAN_POINT('Ctrl Pts',(22.1111871004105,-15.,6.9280356541276));
#32989=CARTESIAN_POINT('Ctrl Pts',(22.1111871004105,-14.75,6.9280356541276));
#32990=CARTESIAN_POINT('Ctrl Pts',(22.3178718686104,-15.,6.69679414480925));
#32991=CARTESIAN_POINT('Ctrl Pts',(22.3178718686104,-14.75,6.69679414480925));
#32992=CARTESIAN_POINT('Ctrl Pts',(22.5122783780098,-15.,6.60061407834291));
#32993=CARTESIAN_POINT('Ctrl Pts',(22.5122783780098,-14.75,6.60061407834291));
#32994=CARTESIAN_POINT('',(22.1111871004105,-14.75,6.9280356541276));
#32995=CARTESIAN_POINT('',(22.1111871004105,-15.,6.9280356541276));
#32996=CARTESIAN_POINT('',(22.5122783780098,-14.75,6.60061407834291));
#32997=CARTESIAN_POINT('Ctrl Pts',(22.1111871004105,-14.75,6.9280356541276));
#32998=CARTESIAN_POINT('Ctrl Pts',(22.3178718686104,-14.75,6.69679414480925));
#32999=CARTESIAN_POINT('Ctrl Pts',(22.5122783780098,-14.75,6.60061407834291));
#33000=CARTESIAN_POINT('',(22.5122783780098,-15.,6.60061407834291));
#33001=CARTESIAN_POINT('Ctrl Pts',(21.7592087090015,-15.,7.46828120201826));
#33002=CARTESIAN_POINT('Ctrl Pts',(21.7592087090015,-14.75,7.46828120201826));
#33003=CARTESIAN_POINT('Ctrl Pts',(21.9045020341873,-15.,7.15927708894014));
#33004=CARTESIAN_POINT('Ctrl Pts',(21.9045020341873,-14.75,7.15927708894014));
#33005=CARTESIAN_POINT('Ctrl Pts',(22.1111871004105,-15.,6.9280356541276));
#33006=CARTESIAN_POINT('Ctrl Pts',(22.1111871004105,-14.75,6.9280356541276));
#33007=CARTESIAN_POINT('',(21.7592087090015,-14.75,7.46828120201826));
#33008=CARTESIAN_POINT('',(21.7592087090015,-15.,7.46828120201826));
#33009=CARTESIAN_POINT('Ctrl Pts',(21.7592087090015,-14.75,7.46828120201826));
#33010=CARTESIAN_POINT('Ctrl Pts',(21.9045020341873,-14.75,7.15927708894014));
#33011=CARTESIAN_POINT('Ctrl Pts',(22.1111871004105,-14.75,6.9280356541276));
#33012=CARTESIAN_POINT('Origin',(21.4031378626823,-15.,7.46828120201826));
#33013=CARTESIAN_POINT('',(21.4031378626823,-14.75,7.46828120201826));
#33014=CARTESIAN_POINT('',(21.4031378626823,-15.,7.46828120201826));
#33015=CARTESIAN_POINT('',(21.4031378626823,-14.75,7.46828120201826));
#33016=CARTESIAN_POINT('Ctrl Pts',(21.5934516191483,-15.,7.080491296947));
#33017=CARTESIAN_POINT('Ctrl Pts',(21.5934516191483,-14.75,7.080491296947));
#33018=CARTESIAN_POINT('Ctrl Pts',(21.4665756821632,-15.,7.29638490825891));
#33019=CARTESIAN_POINT('Ctrl Pts',(21.4665756821632,-14.75,7.29638490825891));
#33020=CARTESIAN_POINT('Ctrl Pts',(21.4031378626823,-15.,7.46828120201826));
#33021=CARTESIAN_POINT('Ctrl Pts',(21.4031378626823,-14.75,7.46828120201826));
#33022=CARTESIAN_POINT('',(21.5934516191483,-14.75,7.080491296947));
#33023=CARTESIAN_POINT('',(21.5934516191483,-15.,7.080491296947));
#33024=CARTESIAN_POINT('Ctrl Pts',(21.5934516191483,-14.75,7.080491296947));
#33025=CARTESIAN_POINT('Ctrl Pts',(21.4665756821632,-14.75,7.29638490825891));
#33026=CARTESIAN_POINT('Ctrl Pts',(21.4031378626823,-14.75,7.46828120201826));
#33027=CARTESIAN_POINT('Ctrl Pts',(21.8472033441067,-15.,6.73158269375563));
#33028=CARTESIAN_POINT('Ctrl Pts',(21.8472033441067,-14.75,6.73158269375563));
#33029=CARTESIAN_POINT('Ctrl Pts',(21.7203274071217,-15.,6.86459768563509));
#33030=CARTESIAN_POINT('Ctrl Pts',(21.7203274071217,-14.75,6.86459768563509));
#33031=CARTESIAN_POINT('Ctrl Pts',(21.5934516191483,-15.,7.080491296947));
#33032=CARTESIAN_POINT('Ctrl Pts',(21.5934516191483,-14.75,7.080491296947));
#33033=CARTESIAN_POINT('',(21.8472033441067,-14.75,6.73158269375563));
#33034=CARTESIAN_POINT('',(21.8472033441067,-15.,6.73158269375563));
#33035=CARTESIAN_POINT('Ctrl Pts',(21.8472033441067,-14.75,6.73158269375563));
#33036=CARTESIAN_POINT('Ctrl Pts',(21.7203274071217,-14.75,6.86459768563509));
#33037=CARTESIAN_POINT('Ctrl Pts',(21.5934516191483,-14.75,7.080491296947));
#33038=CARTESIAN_POINT('Origin',(19.5,-15.,6.73158269375563));
#33039=CARTESIAN_POINT('',(19.5,-14.75,6.73158269375563));
#33040=CARTESIAN_POINT('',(19.5,-15.,6.73158269375563));
#33041=CARTESIAN_POINT('',(19.5,-14.75,6.73158269375563));
#33042=CARTESIAN_POINT('Origin',(19.5,-15.,6.3632333651185));
#33043=CARTESIAN_POINT('',(19.5,-14.75,6.3632333651185));
#33044=CARTESIAN_POINT('',(19.5,-15.,6.3632333651185));
#33045=CARTESIAN_POINT('',(19.5,-14.75,6.3632333651185));
#33046=CARTESIAN_POINT('Origin',(22.5122783780098,-15.,6.3632333651185));
#33047=CARTESIAN_POINT('',(22.5122783780098,-14.75,6.3632333651185));
#33048=CARTESIAN_POINT('',(22.5122783780098,-15.,6.3632333651185));
#33049=CARTESIAN_POINT('',(22.5122783780098,-14.75,6.3632333651185));
#33050=CARTESIAN_POINT('Origin',(22.5122783780098,-15.,6.60061407834291));
#33051=CARTESIAN_POINT('',(22.5122783780098,-14.75,6.60061407834291));
#33052=CARTESIAN_POINT('Origin',(21.0061391890049,-14.75,6.91575728356838));
#33053=CARTESIAN_POINT('Ctrl Pts',(19.9062074422836,-15.,-6.90143261104822));
#33054=CARTESIAN_POINT('Ctrl Pts',(19.9062074422836,-14.75,-6.90143261104822));
#33055=CARTESIAN_POINT('Ctrl Pts',(20.0054569244385,-15.,-7.14699868112802));
#33056=CARTESIAN_POINT('Ctrl Pts',(20.0054569244385,-14.75,-7.14699868112802));
#33057=CARTESIAN_POINT('Ctrl Pts',(20.1180080771446,-15.,-7.27387461811304));
#33058=CARTESIAN_POINT('Ctrl Pts',(20.1180080771446,-14.75,-7.27387461811304));
#33059=CARTESIAN_POINT('',(19.9062074422836,-14.75,-6.90143261104822));
#33060=CARTESIAN_POINT('',(19.9062074422836,-15.,-6.90143261104822));
#33061=CARTESIAN_POINT('',(20.1180080771446,-14.75,-7.27387461811304));
#33062=CARTESIAN_POINT('Ctrl Pts',(19.9062074422836,-14.75,-6.90143261104822));
#33063=CARTESIAN_POINT('Ctrl Pts',(20.0054569244385,-14.75,-7.14699868112802));
#33064=CARTESIAN_POINT('Ctrl Pts',(20.1180080771446,-14.75,-7.27387461811304));
#33065=CARTESIAN_POINT('',(20.1180080771446,-15.,-7.27387461811304));
#33066=CARTESIAN_POINT('Ctrl Pts',(19.8069576621056,-15.,-6.39802191406488));
#33067=CARTESIAN_POINT('Ctrl Pts',(19.8069576621056,-14.75,-6.39802191406488));
#33068=CARTESIAN_POINT('Ctrl Pts',(19.8069576621056,-15.,-6.6558663919568));
#33069=CARTESIAN_POINT('Ctrl Pts',(19.8069576621056,-14.75,-6.6558663919568));
#33070=CARTESIAN_POINT('Ctrl Pts',(19.9062074422836,-15.,-6.90143261104822));
#33071=CARTESIAN_POINT('Ctrl Pts',(19.9062074422836,-14.75,-6.90143261104822));
#33072=CARTESIAN_POINT('',(19.8069576621056,-14.75,-6.39802191406488));
#33073=CARTESIAN_POINT('',(19.8069576621056,-15.,-6.39802191406488));
#33074=CARTESIAN_POINT('Ctrl Pts',(19.8069576621056,-14.75,-6.39802191406488));
#33075=CARTESIAN_POINT('Ctrl Pts',(19.8069576621056,-14.75,-6.6558663919568));
#33076=CARTESIAN_POINT('Ctrl Pts',(19.9062074422836,-14.75,-6.90143261104822));
#33077=CARTESIAN_POINT('Ctrl Pts',(19.9379263520241,-15.,-5.8373125270009));
#33078=CARTESIAN_POINT('Ctrl Pts',(19.9379263520241,-14.75,-5.8373125270009));
#33079=CARTESIAN_POINT('Ctrl Pts',(19.8069576621056,-15.,-6.10129613429308));
#33080=CARTESIAN_POINT('Ctrl Pts',(19.8069576621056,-14.75,-6.10129613429308));
#33081=CARTESIAN_POINT('Ctrl Pts',(19.8069576621056,-15.,-6.39802191406488));
#33082=CARTESIAN_POINT('Ctrl Pts',(19.8069576621056,-14.75,-6.39802191406488));
#33083=CARTESIAN_POINT('',(19.9379263520241,-14.75,-5.8373125270009));
#33084=CARTESIAN_POINT('',(19.9379263520241,-15.,-5.8373125270009));
#33085=CARTESIAN_POINT('Ctrl Pts',(19.9379263520241,-14.75,-5.8373125270009));
#33086=CARTESIAN_POINT('Ctrl Pts',(19.8069576621056,-14.75,-6.10129613429308));
#33087=CARTESIAN_POINT('Ctrl Pts',(19.8069576621056,-14.75,-6.39802191406488));
#33088=CARTESIAN_POINT('Ctrl Pts',(20.3390176296234,-15.,-5.43519791215658));
#33089=CARTESIAN_POINT('Ctrl Pts',(20.3390176296234,-14.75,-5.43519791215658));
#33090=CARTESIAN_POINT('Ctrl Pts',(20.0688950419426,-15.,-5.57332884520292));
#33091=CARTESIAN_POINT('Ctrl Pts',(20.0688950419426,-14.75,-5.57332884520292));
#33092=CARTESIAN_POINT('Ctrl Pts',(19.9379263520241,-15.,-5.8373125270009));
#33093=CARTESIAN_POINT('Ctrl Pts',(19.9379263520241,-14.75,-5.8373125270009));
#33094=CARTESIAN_POINT('',(20.3390176296234,-14.75,-5.43519791215658));
#33095=CARTESIAN_POINT('',(20.3390176296234,-15.,-5.43519791215658));
#33096=CARTESIAN_POINT('Ctrl Pts',(20.3390176296234,-14.75,-5.43519791215658));
#33097=CARTESIAN_POINT('Ctrl Pts',(20.0688950419426,-14.75,-5.57332884520292));
#33098=CARTESIAN_POINT('Ctrl Pts',(19.9379263520241,-14.75,-5.8373125270009));
#33099=CARTESIAN_POINT('Ctrl Pts',(21.0102319419384,-15.,-5.29706697911024));
#33100=CARTESIAN_POINT('Ctrl Pts',(21.0102319419384,-14.75,-5.29706697911024));
#33101=CARTESIAN_POINT('Ctrl Pts',(20.6091405153275,-15.,-5.29706697911024));
#33102=CARTESIAN_POINT('Ctrl Pts',(20.6091405153275,-14.75,-5.29706697911024));
#33103=CARTESIAN_POINT('Ctrl Pts',(20.3390176296234,-15.,-5.43519791215658));
#33104=CARTESIAN_POINT('Ctrl Pts',(20.3390176296234,-14.75,-5.43519791215658));
#33105=CARTESIAN_POINT('',(21.0102319419384,-14.75,-5.29706697911024));
#33106=CARTESIAN_POINT('',(21.0102319419384,-15.,-5.29706697911024));
#33107=CARTESIAN_POINT('Ctrl Pts',(21.0102319419384,-14.75,-5.29706697911024));
#33108=CARTESIAN_POINT('Ctrl Pts',(20.6091405153275,-14.75,-5.29706697911024));
#33109=CARTESIAN_POINT('Ctrl Pts',(20.3390176296234,-14.75,-5.43519791215658));
#33110=CARTESIAN_POINT('Ctrl Pts',(21.6139155328274,-15.,-5.41166450828314));
#33111=CARTESIAN_POINT('Ctrl Pts',(21.6139155328274,-14.75,-5.41166450828314));
#33112=CARTESIAN_POINT('Ctrl Pts',(21.3356071412563,-15.,-5.29706697911024));
#33113=CARTESIAN_POINT('Ctrl Pts',(21.3356071412563,-14.75,-5.29706697911024));
#33114=CARTESIAN_POINT('Ctrl Pts',(21.0102319419384,-15.,-5.29706697911024));
#33115=CARTESIAN_POINT('Ctrl Pts',(21.0102319419384,-14.75,-5.29706697911024));
#33116=CARTESIAN_POINT('',(21.6139155328274,-14.75,-5.41166450828314));
#33117=CARTESIAN_POINT('',(21.6139155328274,-15.,-5.41166450828314));
#33118=CARTESIAN_POINT('Ctrl Pts',(21.6139155328274,-14.75,-5.41166450828314));
#33119=CARTESIAN_POINT('Ctrl Pts',(21.3356071412563,-14.75,-5.29706697911024));
#33120=CARTESIAN_POINT('Ctrl Pts',(21.0102319419384,-14.75,-5.29706697911024));
#33121=CARTESIAN_POINT('Ctrl Pts',(21.9106413125992,-15.,-5.60095507651567));
#33122=CARTESIAN_POINT('Ctrl Pts',(21.9106413125992,-14.75,-5.60095507651567));
#33123=CARTESIAN_POINT('Ctrl Pts',(21.7755798697472,-15.,-5.47919515520334));
#33124=CARTESIAN_POINT('Ctrl Pts',(21.7755798697472,-14.75,-5.47919515520334));
#33125=CARTESIAN_POINT('Ctrl Pts',(21.6139155328274,-15.,-5.41166450828314));
#33126=CARTESIAN_POINT('Ctrl Pts',(21.6139155328274,-14.75,-5.41166450828314));
#33127=CARTESIAN_POINT('',(21.9106413125992,-14.75,-5.60095507651567));
#33128=CARTESIAN_POINT('',(21.9106413125992,-15.,-5.60095507651567));
#33129=CARTESIAN_POINT('Ctrl Pts',(21.9106413125992,-14.75,-5.60095507651567));
#33130=CARTESIAN_POINT('Ctrl Pts',(21.7755798697472,-14.75,-5.47919515520334));
#33131=CARTESIAN_POINT('Ctrl Pts',(21.6139155328274,-14.75,-5.41166450828314));
#33132=CARTESIAN_POINT('Ctrl Pts',(22.128581225872,-15.,-5.92121426016092));
#33133=CARTESIAN_POINT('Ctrl Pts',(22.128581225872,-14.75,-5.92121426016092));
#33134=CARTESIAN_POINT('Ctrl Pts',(22.0457027554512,-15.,-5.7227149233222));
#33135=CARTESIAN_POINT('Ctrl Pts',(22.0457027554512,-14.75,-5.7227149233222));
#33136=CARTESIAN_POINT('Ctrl Pts',(21.9106413125992,-15.,-5.60095507651567));
#33137=CARTESIAN_POINT('Ctrl Pts',(21.9106413125992,-14.75,-5.60095507651567));
#33138=CARTESIAN_POINT('',(22.128581225872,-14.75,-5.92121426016092));
#33139=CARTESIAN_POINT('',(22.128581225872,-15.,-5.92121426016092));
#33140=CARTESIAN_POINT('Ctrl Pts',(22.128581225872,-14.75,-5.92121426016092));
#33141=CARTESIAN_POINT('Ctrl Pts',(22.0457027554512,-14.75,-5.7227149233222));
#33142=CARTESIAN_POINT('Ctrl Pts',(21.9106413125992,-14.75,-5.60095507651567));
#33143=CARTESIAN_POINT('Ctrl Pts',(22.2114599943161,-15.,-6.39188278466463));
#33144=CARTESIAN_POINT('Ctrl Pts',(22.2114599943161,-14.75,-6.39188278466463));
#33145=CARTESIAN_POINT('Ctrl Pts',(22.2114599943161,-15.,-6.11971367150545));
#33146=CARTESIAN_POINT('Ctrl Pts',(22.2114599943161,-14.75,-6.11971367150545));
#33147=CARTESIAN_POINT('Ctrl Pts',(22.128581225872,-15.,-5.92121426016092));
#33148=CARTESIAN_POINT('Ctrl Pts',(22.128581225872,-14.75,-5.92121426016092));
#33149=CARTESIAN_POINT('',(22.2114599943161,-14.75,-6.39188278466463));
#33150=CARTESIAN_POINT('',(22.2114599943161,-15.,-6.39188278466463));
#33151=CARTESIAN_POINT('Ctrl Pts',(22.2114599943161,-14.75,-6.39188278466463));
#33152=CARTESIAN_POINT('Ctrl Pts',(22.2114599943161,-14.75,-6.11971367150545));
#33153=CARTESIAN_POINT('Ctrl Pts',(22.128581225872,-14.75,-5.92121426016092));
#33154=CARTESIAN_POINT('Ctrl Pts',(22.1326739788055,-15.,-6.80525247007608));
#33155=CARTESIAN_POINT('Ctrl Pts',(22.1326739788055,-14.75,-6.80525247007608));
#33156=CARTESIAN_POINT('Ctrl Pts',(22.2114599943161,-15.,-6.61903146654367));
#33157=CARTESIAN_POINT('Ctrl Pts',(22.2114599943161,-14.75,-6.61903146654367));
#33158=CARTESIAN_POINT('Ctrl Pts',(22.2114599943161,-15.,-6.39188278466463));
#33159=CARTESIAN_POINT('Ctrl Pts',(22.2114599943161,-14.75,-6.39188278466463));
#33160=CARTESIAN_POINT('',(22.1326739788055,-14.75,-6.80525247007608));
#33161=CARTESIAN_POINT('',(22.1326739788055,-15.,-6.80525247007608));
#33162=CARTESIAN_POINT('Ctrl Pts',(22.1326739788055,-14.75,-6.80525247007608));
#33163=CARTESIAN_POINT('Ctrl Pts',(22.2114599943161,-14.75,-6.61903146654367));
#33164=CARTESIAN_POINT('Ctrl Pts',(22.2114599943161,-14.75,-6.39188278466463));
#33165=CARTESIAN_POINT('Ctrl Pts',(21.9229195713997,-15.,-7.09174636751413));
#33166=CARTESIAN_POINT('Ctrl Pts',(21.9229195713997,-14.75,-7.09174636751413));
#33167=CARTESIAN_POINT('Ctrl Pts',(22.0538882613182,-15.,-6.99147347360849));
#33168=CARTESIAN_POINT('Ctrl Pts',(22.0538882613182,-14.75,-6.99147347360849));
#33169=CARTESIAN_POINT('Ctrl Pts',(22.1326739788055,-15.,-6.80525247007608));
#33170=CARTESIAN_POINT('Ctrl Pts',(22.1326739788055,-14.75,-6.80525247007608));
#33171=CARTESIAN_POINT('',(21.9229195713997,-14.75,-7.09174636751413));
#33172=CARTESIAN_POINT('',(21.9229195713997,-15.,-7.09174636751413));
#33173=CARTESIAN_POINT('Ctrl Pts',(21.9229195713997,-14.75,-7.09174636751413));
#33174=CARTESIAN_POINT('Ctrl Pts',(22.0538882613182,-14.75,-6.99147347360849));
#33175=CARTESIAN_POINT('Ctrl Pts',(22.1326739788055,-14.75,-6.80525247007608));
#33176=CARTESIAN_POINT('Ctrl Pts',(21.562755972147,-15.,-7.25955013185739));
#33177=CARTESIAN_POINT('Ctrl Pts',(21.562755972147,-14.75,-7.25955013185739));
#33178=CARTESIAN_POINT('Ctrl Pts',(21.7919510304928,-15.,-7.19201926141977));
#33179=CARTESIAN_POINT('Ctrl Pts',(21.7919510304928,-14.75,-7.19201926141977));
#33180=CARTESIAN_POINT('Ctrl Pts',(21.9229195713997,-15.,-7.09174636751413));
#33181=CARTESIAN_POINT('Ctrl Pts',(21.9229195713997,-14.75,-7.09174636751413));
#33182=CARTESIAN_POINT('',(21.562755972147,-14.75,-7.25955013185739));
#33183=CARTESIAN_POINT('',(21.562755972147,-15.,-7.25955013185739));
#33184=CARTESIAN_POINT('Ctrl Pts',(21.562755972147,-14.75,-7.25955013185739));
#33185=CARTESIAN_POINT('Ctrl Pts',(21.7919510304928,-14.75,-7.19201926141977));
#33186=CARTESIAN_POINT('Ctrl Pts',(21.9229195713997,-14.75,-7.09174636751413));
#33187=CARTESIAN_POINT('Origin',(21.6609823405743,-15.,-7.61766735464334));
#33188=CARTESIAN_POINT('',(21.6609823405743,-14.75,-7.61766735464334));
#33189=CARTESIAN_POINT('',(21.6609823405743,-15.,-7.61766735464334));
#33190=CARTESIAN_POINT('',(21.6609823405743,-14.75,-7.61766735464334));
#33191=CARTESIAN_POINT('Ctrl Pts',(22.1521146297455,-15.,-7.39051882177591));
#33192=CARTESIAN_POINT('Ctrl Pts',(22.1521146297455,-14.75,-7.39051882177591));
#33193=CARTESIAN_POINT('Ctrl Pts',(21.9638473987579,-15.,-7.53990475088358));
#33194=CARTESIAN_POINT('Ctrl Pts',(21.9638473987579,-14.75,-7.53990475088358));
#33195=CARTESIAN_POINT('Ctrl Pts',(21.6609823405743,-15.,-7.61766735464334));
#33196=CARTESIAN_POINT('Ctrl Pts',(21.6609823405743,-14.75,-7.61766735464334));
#33197=CARTESIAN_POINT('',(22.1521146297455,-14.75,-7.39051882177591));
#33198=CARTESIAN_POINT('',(22.1521146297455,-15.,-7.39051882177591));
#33199=CARTESIAN_POINT('Ctrl Pts',(22.1521146297455,-14.75,-7.39051882177591));
#33200=CARTESIAN_POINT('Ctrl Pts',(21.9638473987579,-14.75,-7.53990475088358));
#33201=CARTESIAN_POINT('Ctrl Pts',(21.6609823405743,-14.75,-7.61766735464334));
#33202=CARTESIAN_POINT('Ctrl Pts',(22.445770919323,-15.,-6.9781719520688));
#33203=CARTESIAN_POINT('Ctrl Pts',(22.445770919323,-14.75,-6.9781719520688));
#33204=CARTESIAN_POINT('Ctrl Pts',(22.3403821587563,-15.,-7.24113259464502));
#33205=CARTESIAN_POINT('Ctrl Pts',(22.3403821587563,-14.75,-7.24113259464502));
#33206=CARTESIAN_POINT('Ctrl Pts',(22.1521146297455,-15.,-7.39051882177591));
#33207=CARTESIAN_POINT('Ctrl Pts',(22.1521146297455,-14.75,-7.39051882177591));
#33208=CARTESIAN_POINT('',(22.445770919323,-14.75,-6.9781719520688));
#33209=CARTESIAN_POINT('',(22.445770919323,-15.,-6.9781719520688));
#33210=CARTESIAN_POINT('Ctrl Pts',(22.445770919323,-14.75,-6.9781719520688));
#33211=CARTESIAN_POINT('Ctrl Pts',(22.3403821587563,-14.75,-7.24113259464502));
#33212=CARTESIAN_POINT('Ctrl Pts',(22.1521146297455,-14.75,-7.39051882177591));
#33213=CARTESIAN_POINT('Ctrl Pts',(22.5511596798897,-15.,-6.38983640819788));
#33214=CARTESIAN_POINT('Ctrl Pts',(22.5511596798897,-14.75,-6.38983640819788));
#33215=CARTESIAN_POINT('Ctrl Pts',(22.5511596798897,-15.,-6.71521160751581));
#33216=CARTESIAN_POINT('Ctrl Pts',(22.5511596798897,-14.75,-6.71521160751581));
#33217=CARTESIAN_POINT('Ctrl Pts',(22.445770919323,-15.,-6.9781719520688));
#33218=CARTESIAN_POINT('Ctrl Pts',(22.445770919323,-14.75,-6.9781719520688));
#33219=CARTESIAN_POINT('',(22.5511596798897,-14.75,-6.38983640819788));
#33220=CARTESIAN_POINT('',(22.5511596798897,-15.,-6.38983640819788));
#33221=CARTESIAN_POINT('Ctrl Pts',(22.5511596798897,-14.75,-6.38983640819788));
#33222=CARTESIAN_POINT('Ctrl Pts',(22.5511596798897,-14.75,-6.71521160751581));
#33223=CARTESIAN_POINT('Ctrl Pts',(22.445770919323,-14.75,-6.9781719520688));
#33224=CARTESIAN_POINT('Ctrl Pts',(22.3669852018356,-15.,-5.59788551181555));
#33225=CARTESIAN_POINT('Ctrl Pts',(22.3669852018356,-14.75,-5.59788551181555));
#33226=CARTESIAN_POINT('Ctrl Pts',(22.5511596798897,-15.,-5.94167817384004));
#33227=CARTESIAN_POINT('Ctrl Pts',(22.5511596798897,-14.75,-5.94167817384004));
#33228=CARTESIAN_POINT('Ctrl Pts',(22.5511596798897,-15.,-6.38983640819788));
#33229=CARTESIAN_POINT('Ctrl Pts',(22.5511596798897,-14.75,-6.38983640819788));
#33230=CARTESIAN_POINT('',(22.3669852018356,-14.75,-5.59788551181555));
#33231=CARTESIAN_POINT('',(22.3669852018356,-15.,-5.59788551181555));
#33232=CARTESIAN_POINT('Ctrl Pts',(22.3669852018356,-14.75,-5.59788551181555));
#33233=CARTESIAN_POINT('Ctrl Pts',(22.5511596798897,-14.75,-5.94167817384004));
#33234=CARTESIAN_POINT('Ctrl Pts',(22.5511596798897,-14.75,-6.38983640819788));
#33235=CARTESIAN_POINT('Ctrl Pts',(21.8032061755657,-15.,-5.07094141095877));
#33236=CARTESIAN_POINT('Ctrl Pts',(21.8032061755657,-14.75,-5.07094141095877));
#33237=CARTESIAN_POINT('Ctrl Pts',(22.1828104257584,-15.,-5.25409284979105));
#33238=CARTESIAN_POINT('Ctrl Pts',(22.1828104257584,-14.75,-5.25409284979105));
#33239=CARTESIAN_POINT('Ctrl Pts',(22.3669852018356,-15.,-5.59788551181555));
#33240=CARTESIAN_POINT('Ctrl Pts',(22.3669852018356,-14.75,-5.59788551181555));
#33241=CARTESIAN_POINT('',(21.8032061755657,-14.75,-5.07094141095877));
#33242=CARTESIAN_POINT('',(21.8032061755657,-15.,-5.07094141095877));
#33243=CARTESIAN_POINT('Ctrl Pts',(21.8032061755657,-14.75,-5.07094141095877));
#33244=CARTESIAN_POINT('Ctrl Pts',(22.1828104257584,-14.75,-5.25409284979105));
#33245=CARTESIAN_POINT('Ctrl Pts',(22.3669852018356,-14.75,-5.59788551181555));
#33246=CARTESIAN_POINT('Ctrl Pts',(20.9856754243374,-15.,-4.88778999075293));
#33247=CARTESIAN_POINT('Ctrl Pts',(20.9856754243374,-14.75,-4.88778999075293));
#33248=CARTESIAN_POINT('Ctrl Pts',(21.4236017763615,-15.,-4.88778999075293));
#33249=CARTESIAN_POINT('Ctrl Pts',(21.4236017763615,-14.75,-4.88778999075293));
#33250=CARTESIAN_POINT('Ctrl Pts',(21.8032061755657,-15.,-5.07094141095877));
#33251=CARTESIAN_POINT('Ctrl Pts',(21.8032061755657,-14.75,-5.07094141095877));
#33252=CARTESIAN_POINT('',(20.9856754243374,-14.75,-4.88778999075293));
#33253=CARTESIAN_POINT('',(20.9856754243374,-15.,-4.88778999075293));
#33254=CARTESIAN_POINT('Ctrl Pts',(20.9856754243374,-14.75,-4.88778999075293));
#33255=CARTESIAN_POINT('Ctrl Pts',(21.4236017763615,-14.75,-4.88778999075293));
#33256=CARTESIAN_POINT('Ctrl Pts',(21.8032061755657,-14.75,-5.07094141095877));
#33257=CARTESIAN_POINT('Ctrl Pts',(20.1855389475822,-15.,-5.07196459919214));
#33258=CARTESIAN_POINT('Ctrl Pts',(20.1855389475822,-14.75,-5.07196459919214));
#33259=CARTESIAN_POINT('Ctrl Pts',(20.5436561703682,-15.,-4.88778999075293));
#33260=CARTESIAN_POINT('Ctrl Pts',(20.5436561703682,-14.75,-4.88778999075293));
#33261=CARTESIAN_POINT('Ctrl Pts',(20.9856754243374,-15.,-4.88778999075293));
#33262=CARTESIAN_POINT('Ctrl Pts',(20.9856754243374,-14.75,-4.88778999075293));
#33263=CARTESIAN_POINT('',(20.1855389475822,-14.75,-5.07196459919214));
#33264=CARTESIAN_POINT('',(20.1855389475822,-15.,-5.07196459919214));
#33265=CARTESIAN_POINT('Ctrl Pts',(20.1855389475822,-14.75,-5.07196459919214));
#33266=CARTESIAN_POINT('Ctrl Pts',(20.5436561703682,-14.75,-4.88778999075293));
#33267=CARTESIAN_POINT('Ctrl Pts',(20.9856754243374,-14.75,-4.88778999075293));
#33268=CARTESIAN_POINT('Ctrl Pts',(19.638131082058,-15.,-5.61732616275549));
#33269=CARTESIAN_POINT('Ctrl Pts',(19.638131082058,-14.75,-5.61732616275549));
#33270=CARTESIAN_POINT('Ctrl Pts',(19.8274214267731,-15.,-5.2561392262578));
#33271=CARTESIAN_POINT('Ctrl Pts',(19.8274214267731,-14.75,-5.2561392262578));
#33272=CARTESIAN_POINT('Ctrl Pts',(20.1855389475822,-15.,-5.07196459919214));
#33273=CARTESIAN_POINT('Ctrl Pts',(20.1855389475822,-14.75,-5.07196459919214));
#33274=CARTESIAN_POINT('',(19.638131082058,-14.75,-5.61732616275549));
#33275=CARTESIAN_POINT('',(19.638131082058,-15.,-5.61732616275549));
#33276=CARTESIAN_POINT('Ctrl Pts',(19.638131082058,-14.75,-5.61732616275549));
#33277=CARTESIAN_POINT('Ctrl Pts',(19.8274214267731,-14.75,-5.2561392262578));
#33278=CARTESIAN_POINT('Ctrl Pts',(20.1855389475822,-14.75,-5.07196459919214));
#33279=CARTESIAN_POINT('Ctrl Pts',(19.4488404393196,-15.,-6.42053220421076));
#33280=CARTESIAN_POINT('Ctrl Pts',(19.4488404393196,-14.75,-6.42053220421076));
#33281=CARTESIAN_POINT('Ctrl Pts',(19.4488404393196,-15.,-5.97851309925318));
#33282=CARTESIAN_POINT('Ctrl Pts',(19.4488404393196,-14.75,-5.97851309925318));
#33283=CARTESIAN_POINT('Ctrl Pts',(19.638131082058,-15.,-5.61732616275549));
#33284=CARTESIAN_POINT('Ctrl Pts',(19.638131082058,-14.75,-5.61732616275549));
#33285=CARTESIAN_POINT('',(19.4488404393196,-14.75,-6.42053220421076));
#33286=CARTESIAN_POINT('',(19.4488404393196,-15.,-6.42053220421076));
#33287=CARTESIAN_POINT('Ctrl Pts',(19.4488404393196,-14.75,-6.42053220421076));
#33288=CARTESIAN_POINT('Ctrl Pts',(19.4488404393196,-14.75,-5.97851309925318));
#33289=CARTESIAN_POINT('Ctrl Pts',(19.638131082058,-14.75,-5.61732616275549));
#33290=CARTESIAN_POINT('Ctrl Pts',(19.5665074586868,-15.,-7.0590041950345));
#33291=CARTESIAN_POINT('Ctrl Pts',(19.5665074586868,-14.75,-7.0590041950345));
#33292=CARTESIAN_POINT('Ctrl Pts',(19.4488404393196,-15.,-6.74795377999544));
#33293=CARTESIAN_POINT('Ctrl Pts',(19.4488404393196,-14.75,-6.74795377999544));
#33294=CARTESIAN_POINT('Ctrl Pts',(19.4488404393196,-15.,-6.42053220421076));
#33295=CARTESIAN_POINT('Ctrl Pts',(19.4488404393196,-14.75,-6.42053220421076));
#33296=CARTESIAN_POINT('',(19.5665074586868,-14.75,-7.0590041950345));
#33297=CARTESIAN_POINT('',(19.5665074586868,-15.,-7.0590041950345));
#33298=CARTESIAN_POINT('Ctrl Pts',(19.5665074586868,-14.75,-7.0590041950345));
#33299=CARTESIAN_POINT('Ctrl Pts',(19.4488404393196,-14.75,-6.74795377999544));
#33300=CARTESIAN_POINT('Ctrl Pts',(19.4488404393196,-14.75,-6.42053220421076));
#33301=CARTESIAN_POINT('Ctrl Pts',(19.9174625873566,-15.,-7.66268793493509));
#33302=CARTESIAN_POINT('Ctrl Pts',(19.9174625873566,-14.75,-7.66268793493509));
#33303=CARTESIAN_POINT('Ctrl Pts',(19.684174478054,-15.,-7.37005475908518));
#33304=CARTESIAN_POINT('Ctrl Pts',(19.684174478054,-14.75,-7.37005475908518));
#33305=CARTESIAN_POINT('Ctrl Pts',(19.5665074586868,-15.,-7.0590041950345));
#33306=CARTESIAN_POINT('Ctrl Pts',(19.5665074586868,-14.75,-7.0590041950345));
#33307=CARTESIAN_POINT('',(19.9174625873566,-14.75,-7.66268793493509));
#33308=CARTESIAN_POINT('',(19.9174625873566,-15.,-7.66268793493509));
#33309=CARTESIAN_POINT('Ctrl Pts',(19.9174625873566,-14.75,-7.66268793493509));
#33310=CARTESIAN_POINT('Ctrl Pts',(19.684174478054,-14.75,-7.37005475908518));
#33311=CARTESIAN_POINT('Ctrl Pts',(19.5665074586868,-14.75,-7.0590041950345));
#33312=CARTESIAN_POINT('Origin',(21.0306958556175,-15.,-7.66268793493509));
#33313=CARTESIAN_POINT('',(21.0306958556175,-14.75,-7.66268793493509));
#33314=CARTESIAN_POINT('',(21.0306958556175,-15.,-7.66268793493509));
#33315=CARTESIAN_POINT('',(21.0306958556175,-14.75,-7.66268793493509));
#33316=CARTESIAN_POINT('Origin',(21.0286494791508,-15.,-6.39188278466463));
#33317=CARTESIAN_POINT('',(21.0286494791508,-14.75,-6.39188278466463));
#33318=CARTESIAN_POINT('',(21.0286494791508,-15.,-6.39188278466463));
#33319=CARTESIAN_POINT('',(21.0286494791508,-14.75,-6.39188278466463));
#33320=CARTESIAN_POINT('Origin',(20.6766710877419,-15.,-6.39188278466463));
#33321=CARTESIAN_POINT('',(20.6766710877419,-14.75,-6.39188278466463));
#33322=CARTESIAN_POINT('',(20.6766710877419,-15.,-6.39188278466463));
#33323=CARTESIAN_POINT('',(20.6766710877419,-14.75,-6.39188278466463));
#33324=CARTESIAN_POINT('Origin',(20.6766710877419,-15.,-7.27387461811304));
#33325=CARTESIAN_POINT('',(20.6766710877419,-14.75,-7.27387461811304));
#33326=CARTESIAN_POINT('',(20.6766710877419,-15.,-7.27387461811304));
#33327=CARTESIAN_POINT('',(20.6766710877419,-14.75,-7.27387461811304));
#33328=CARTESIAN_POINT('Origin',(20.1180080771446,-15.,-7.27387461811304));
#33329=CARTESIAN_POINT('',(20.1180080771446,-14.75,-7.27387461811304));
#33330=CARTESIAN_POINT('Origin',(21.0000000596046,-14.75,-6.27523896284401));
#33331=CARTESIAN_POINT('Origin',(15.5,-15.,-18.5));
#33332=CARTESIAN_POINT('',(8.91666666666667,8.4166666666667,-11.9166666666667));
#33333=CARTESIAN_POINT('',(22.5,8.00000000000003,-25.5));
#33334=CARTESIAN_POINT('Origin',(15.25,14.75,-9.5));
#33335=CARTESIAN_POINT('',(5.74999999999999,5.25000000000004,8.74999999999999));
#33336=CARTESIAN_POINT('Origin',(27.,14.75,-18.75));
#33337=CARTESIAN_POINT('Origin',(31.,-15.,-3.46410161513775));
#33338=CARTESIAN_POINT('',(28.,-15.,-1.73205080756888));
#33339=CARTESIAN_POINT('Origin',(15.5,-15.,18.5));
#33340=CARTESIAN_POINT('Origin',(28.,-15.,1.73205080756888));
#33341=CARTESIAN_POINT('',(28.,-15.,1.73205080756888));
#33342=CARTESIAN_POINT('Origin',(28.,-15.,-1.73205080756888));
#45201=UNCERTAINTY_MEASURE_WITH_UNIT(LENGTH_MEASURE(0.01),#45237,
'DISTANCE_ACCURACY_VALUE',
'Maximum model space distance between geometric entities at asserted c
onnectivities');
#45214=UNCERTAINTY_MEASURE_WITH_UNIT(LENGTH_MEASURE(0.01),#45237,
'DISTANCE_ACCURACY_VALUE',
'Maximum model space distance between geometric entities at asserted c
onnectivities');
#45223=(
GEOMETRIC_REPRESENTATION_CONTEXT(3)
GLOBAL_UNCERTAINTY_ASSIGNED_CONTEXT((#45201))
GLOBAL_UNIT_ASSIGNED_CONTEXT((#45237,#45239,#45240))
REPRESENTATION_CONTEXT('','3D')
);
#45236=(
GEOMETRIC_REPRESENTATION_CONTEXT(3)
GLOBAL_UNCERTAINTY_ASSIGNED_CONTEXT((#45214))
GLOBAL_UNIT_ASSIGNED_CONTEXT((#45237,#45239,#45240))
REPRESENTATION_CONTEXT('','3D')
);
#45237=(
LENGTH_UNIT()
NAMED_UNIT(*)
SI_UNIT(.MILLI.,.METRE.)
);
#45239=(
NAMED_UNIT(*)
PLANE_ANGLE_UNIT()
SI_UNIT($,.RADIAN.)
);
#45240=(
NAMED_UNIT(*)
SI_UNIT($,.STERADIAN.)
SOLID_ANGLE_UNIT()
);
#45249=SHAPE_DEFINITION_REPRESENTATION(#45270,#45321);
#45270=PRODUCT_DEFINITION_SHAPE('',$,#45343);
#45321=SHAPE_REPRESENTATION('',(#17175),#45223);
#45334=PRODUCT_DEFINITION_CONTEXT('part definition',#45399,'design');
#45343=PRODUCT_DEFINITION('2026-10-25-23-38-17-681',
'08_Crimping_Die_10_AWG',#45364,#45334);
#45364=PRODUCT_DEFINITION_FORMATION('',$,#45409);
#45399=APPLICATION_CONTEXT(
'Core Data for Automotive Mechanical Design Process');
#45400=PRODUCT_CONTEXT('part definition',#45399,'mechanical');
#45409=PRODUCT('2026-10-25-23-38-17-681','08_Crimping_Die_10_AWG',$,(#45400));
#45471=COLOUR_RGB('Sky Blue',0.24,0.69,0.87);
#45472=FILL_AREA_STYLE_COLOUR('',#45471);
#45473=FILL_AREA_STYLE('',(#45472));
#45474=SURFACE_STYLE_FILL_AREA(#45473);
#45475=SURFACE_SIDE_STYLE('',(#45474));
#45476=SURFACE_STYLE_USAGE(.BOTH.,#45475);
#45477=PRESENTATION_STYLE_ASSIGNMENT((#45476));
ENDSEC;
END-ISO-10303-21;
